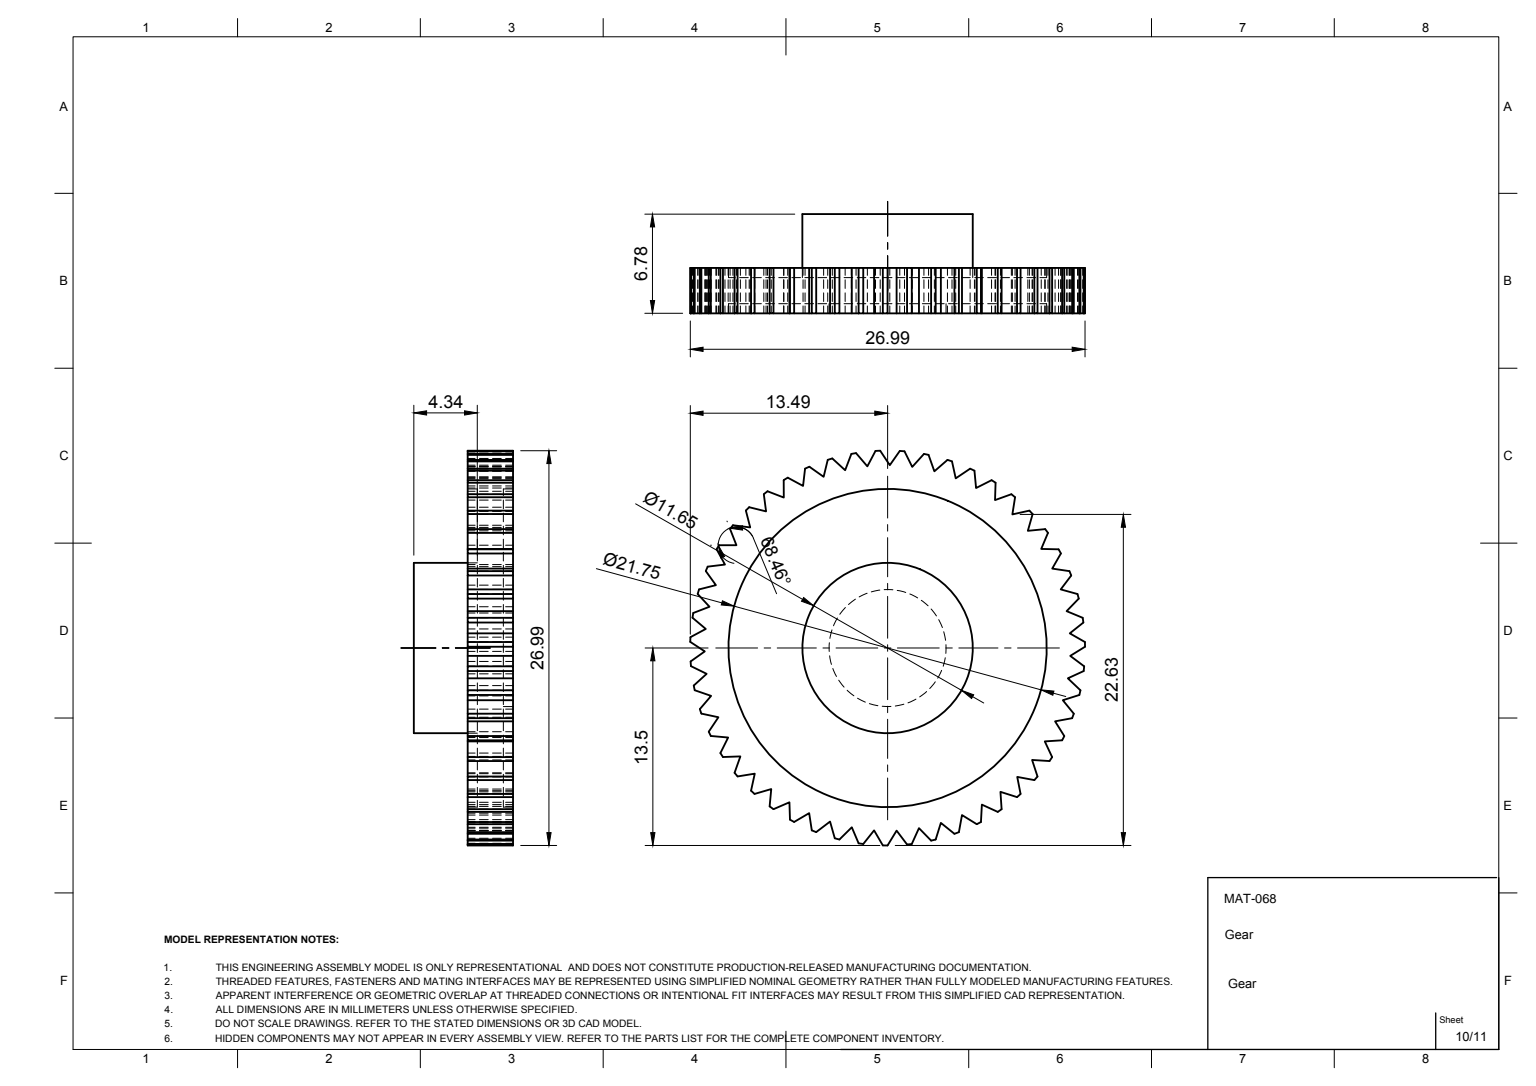
ISO-10303-21;
HEADER;
/* Generated by software containing ST-Developer
 * from STEP Tools, Inc. (www.steptools.com) 
 */

FILE_DESCRIPTION(
/* description */ ('CAx-IF Rec.Pracs.---Representation and Presentation of Product Manufa
cturing Information (PMI)---4.0---2014-10-13'),
/* implementation_level */ '2;1');

FILE_NAME(
/* name */ 'Gear.step',
/* time_stamp */ '2026-10-24T16:53:48-07:00',
/* author */ (''),
/* organization */ (''),
/* preprocessor_version */ 'ST-DEVELOPER v20.2',
/* originating_system */ 'Autodesk Translation Framework v15.17.0.0',
/* authorisation */ '');

FILE_SCHEMA (('AP242_MANAGED_MODEL_BASED_3D_ENGINEERING_MIM_LF { 1 0 10303 442 2 1 4 }'));
ENDSEC;

DATA;
#10=MECHANICAL_DESIGN_GEOMETRIC_PRESENTATION_REPRESENTATION('',(#3497),#107910);
#3477=SHAPE_REPRESENTATION_RELATIONSHIP('SRR','None',#107955,#3487);
#3487=ADVANCED_BREP_SHAPE_REPRESENTATION('',(#3507),#107908);
#3497=STYLED_ITEM('',(#108006),#3507);
#3507=MANIFOLD_SOLID_BREP('Body1',#45545);
#3519=FACE_BOUND('',#9399,.T.);
#3520=FACE_BOUND('',#9401,.T.);
#3521=FACE_BOUND('',#9403,.T.);
#3522=FACE_BOUND('',#9405,.T.);
#3574=PLANE('',#50065);
#3575=PLANE('',#50066);
#3576=PLANE('',#50067);
#3577=PLANE('',#50068);
#3578=PLANE('',#50069);
#3579=PLANE('',#50070);
#3580=PLANE('',#50071);
#3581=PLANE('',#50072);
#3582=PLANE('',#50073);
#3583=PLANE('',#50074);
#3584=PLANE('',#50075);
#3585=PLANE('',#50076);
#3586=PLANE('',#50077);
#3587=PLANE('',#50078);
#3588=PLANE('',#50079);
#3589=PLANE('',#50080);
#3590=PLANE('',#50081);
#3591=PLANE('',#50082);
#3592=PLANE('',#50083);
#3593=PLANE('',#50084);
#3594=PLANE('',#50085);
#3595=PLANE('',#50086);
#3596=PLANE('',#50087);
#3597=PLANE('',#50088);
#3598=PLANE('',#50089);
#3599=PLANE('',#50090);
#3600=PLANE('',#50091);
#3601=PLANE('',#50092);
#3602=PLANE('',#50093);
#3603=PLANE('',#50094);
#3604=PLANE('',#50095);
#3605=PLANE('',#50096);
#3606=PLANE('',#50097);
#3607=PLANE('',#50098);
#3608=PLANE('',#50099);
#3609=PLANE('',#50100);
#3610=PLANE('',#50101);
#3611=PLANE('',#50102);
#3612=PLANE('',#50103);
#3613=PLANE('',#50104);
#3614=PLANE('',#50105);
#3615=PLANE('',#50106);
#3616=PLANE('',#50107);
#3617=PLANE('',#50108);
#3618=PLANE('',#50109);
#3619=PLANE('',#50110);
#3620=PLANE('',#50111);
#3621=PLANE('',#50112);
#3622=PLANE('',#50113);
#3623=PLANE('',#50114);
#3624=PLANE('',#50115);
#3625=PLANE('',#50116);
#3626=PLANE('',#50117);
#3627=PLANE('',#50118);
#3628=PLANE('',#50119);
#3629=PLANE('',#50120);
#3630=PLANE('',#50121);
#3631=PLANE('',#50122);
#3632=PLANE('',#50123);
#3633=PLANE('',#50124);
#3634=PLANE('',#50125);
#3635=PLANE('',#50126);
#3636=PLANE('',#50127);
#3637=PLANE('',#50128);
#3638=PLANE('',#50129);
#3639=PLANE('',#50130);
#3640=PLANE('',#50131);
#3641=PLANE('',#50132);
#3642=PLANE('',#50133);
#3643=PLANE('',#50134);
#3644=PLANE('',#50135);
#3645=PLANE('',#50136);
#3646=PLANE('',#50137);
#3647=PLANE('',#50138);
#3648=PLANE('',#50139);
#3649=PLANE('',#50140);
#3650=PLANE('',#50141);
#3651=PLANE('',#50142);
#3652=PLANE('',#50143);
#3653=PLANE('',#50144);
#3654=PLANE('',#50145);
#3655=PLANE('',#50146);
#3656=PLANE('',#50147);
#3657=PLANE('',#50148);
#3658=PLANE('',#50149);
#3659=PLANE('',#50150);
#3660=PLANE('',#50151);
#3661=PLANE('',#50152);
#3662=PLANE('',#50153);
#3663=PLANE('',#50154);
#3664=PLANE('',#50155);
#3665=PLANE('',#50156);
#3666=PLANE('',#50157);
#3667=PLANE('',#50158);
#3668=PLANE('',#50159);
#3669=PLANE('',#50160);
#3670=PLANE('',#50161);
#3671=PLANE('',#50162);
#3672=PLANE('',#50163);
#3673=PLANE('',#50164);
#3674=PLANE('',#50165);
#3675=PLANE('',#50166);
#3676=PLANE('',#50167);
#3677=PLANE('',#50168);
#3678=PLANE('',#50169);
#3679=PLANE('',#50170);
#3680=PLANE('',#50171);
#3681=PLANE('',#50172);
#6409=FACE_OUTER_BOUND('',#9343,.T.);
#6410=FACE_OUTER_BOUND('',#9344,.T.);
#6411=FACE_OUTER_BOUND('',#9345,.T.);
#6412=FACE_OUTER_BOUND('',#9346,.T.);
#6413=FACE_OUTER_BOUND('',#9347,.T.);
#6414=FACE_OUTER_BOUND('',#9348,.T.);
#6415=FACE_OUTER_BOUND('',#9349,.T.);
#6416=FACE_OUTER_BOUND('',#9350,.T.);
#6417=FACE_OUTER_BOUND('',#9351,.T.);
#6418=FACE_OUTER_BOUND('',#9352,.T.);
#6419=FACE_OUTER_BOUND('',#9353,.T.);
#6420=FACE_OUTER_BOUND('',#9354,.T.);
#6421=FACE_OUTER_BOUND('',#9355,.T.);
#6422=FACE_OUTER_BOUND('',#9356,.T.);
#6423=FACE_OUTER_BOUND('',#9357,.T.);
#6424=FACE_OUTER_BOUND('',#9358,.T.);
#6425=FACE_OUTER_BOUND('',#9359,.T.);
#6426=FACE_OUTER_BOUND('',#9360,.T.);
#6427=FACE_OUTER_BOUND('',#9361,.T.);
#6428=FACE_OUTER_BOUND('',#9362,.T.);
#6429=FACE_OUTER_BOUND('',#9363,.T.);
#6430=FACE_OUTER_BOUND('',#9364,.T.);
#6431=FACE_OUTER_BOUND('',#9365,.T.);
#6432=FACE_OUTER_BOUND('',#9366,.T.);
#6433=FACE_OUTER_BOUND('',#9367,.T.);
#6434=FACE_OUTER_BOUND('',#9368,.T.);
#6435=FACE_OUTER_BOUND('',#9369,.T.);
#6436=FACE_OUTER_BOUND('',#9370,.T.);
#6437=FACE_OUTER_BOUND('',#9371,.T.);
#6438=FACE_OUTER_BOUND('',#9372,.T.);
#6439=FACE_OUTER_BOUND('',#9373,.T.);
#6440=FACE_OUTER_BOUND('',#9374,.T.);
#6441=FACE_OUTER_BOUND('',#9375,.T.);
#6442=FACE_OUTER_BOUND('',#9376,.T.);
#6443=FACE_OUTER_BOUND('',#9377,.T.);
#6444=FACE_OUTER_BOUND('',#9378,.T.);
#6445=FACE_OUTER_BOUND('',#9379,.T.);
#6446=FACE_OUTER_BOUND('',#9380,.T.);
#6447=FACE_OUTER_BOUND('',#9381,.T.);
#6448=FACE_OUTER_BOUND('',#9382,.T.);
#6449=FACE_OUTER_BOUND('',#9383,.T.);
#6450=FACE_OUTER_BOUND('',#9384,.T.);
#6451=FACE_OUTER_BOUND('',#9385,.T.);
#6452=FACE_OUTER_BOUND('',#9386,.T.);
#6453=FACE_OUTER_BOUND('',#9387,.T.);
#6454=FACE_OUTER_BOUND('',#9388,.T.);
#6455=FACE_OUTER_BOUND('',#9389,.T.);
#6456=FACE_OUTER_BOUND('',#9390,.T.);
#6457=FACE_OUTER_BOUND('',#9391,.T.);
#6458=FACE_OUTER_BOUND('',#9392,.T.);
#6459=FACE_OUTER_BOUND('',#9393,.T.);
#6460=FACE_OUTER_BOUND('',#9394,.T.);
#6461=FACE_OUTER_BOUND('',#9395,.T.);
#6462=FACE_OUTER_BOUND('',#9396,.T.);
#6463=FACE_OUTER_BOUND('',#9397,.T.);
#6464=FACE_OUTER_BOUND('',#9398,.T.);
#6465=FACE_OUTER_BOUND('',#9400,.T.);
#6466=FACE_OUTER_BOUND('',#9402,.T.);
#6467=FACE_OUTER_BOUND('',#9404,.T.);
#6468=FACE_OUTER_BOUND('',#9406,.T.);
#6469=FACE_OUTER_BOUND('',#9407,.T.);
#6470=FACE_OUTER_BOUND('',#9408,.T.);
#6471=FACE_OUTER_BOUND('',#9409,.T.);
#6472=FACE_OUTER_BOUND('',#9410,.T.);
#6473=FACE_OUTER_BOUND('',#9411,.T.);
#6474=FACE_OUTER_BOUND('',#9412,.T.);
#6475=FACE_OUTER_BOUND('',#9413,.T.);
#6476=FACE_OUTER_BOUND('',#9414,.T.);
#6477=FACE_OUTER_BOUND('',#9415,.T.);
#6478=FACE_OUTER_BOUND('',#9416,.T.);
#6479=FACE_OUTER_BOUND('',#9417,.T.);
#6480=FACE_OUTER_BOUND('',#9418,.T.);
#6481=FACE_OUTER_BOUND('',#9419,.T.);
#6482=FACE_OUTER_BOUND('',#9420,.T.);
#6483=FACE_OUTER_BOUND('',#9421,.T.);
#6484=FACE_OUTER_BOUND('',#9422,.T.);
#6485=FACE_OUTER_BOUND('',#9423,.T.);
#6486=FACE_OUTER_BOUND('',#9424,.T.);
#6487=FACE_OUTER_BOUND('',#9425,.T.);
#6488=FACE_OUTER_BOUND('',#9426,.T.);
#6489=FACE_OUTER_BOUND('',#9427,.T.);
#6490=FACE_OUTER_BOUND('',#9428,.T.);
#6491=FACE_OUTER_BOUND('',#9429,.T.);
#6492=FACE_OUTER_BOUND('',#9430,.T.);
#6493=FACE_OUTER_BOUND('',#9431,.T.);
#6494=FACE_OUTER_BOUND('',#9432,.T.);
#6495=FACE_OUTER_BOUND('',#9433,.T.);
#6496=FACE_OUTER_BOUND('',#9434,.T.);
#6497=FACE_OUTER_BOUND('',#9435,.T.);
#6498=FACE_OUTER_BOUND('',#9436,.T.);
#6499=FACE_OUTER_BOUND('',#9437,.T.);
#6500=FACE_OUTER_BOUND('',#9438,.T.);
#6501=FACE_OUTER_BOUND('',#9439,.T.);
#6502=FACE_OUTER_BOUND('',#9440,.T.);
#6503=FACE_OUTER_BOUND('',#9441,.T.);
#6504=FACE_OUTER_BOUND('',#9442,.T.);
#6505=FACE_OUTER_BOUND('',#9443,.T.);
#6506=FACE_OUTER_BOUND('',#9444,.T.);
#6507=FACE_OUTER_BOUND('',#9445,.T.);
#6508=FACE_OUTER_BOUND('',#9446,.T.);
#6509=FACE_OUTER_BOUND('',#9447,.T.);
#6510=FACE_OUTER_BOUND('',#9448,.T.);
#6511=FACE_OUTER_BOUND('',#9449,.T.);
#6512=FACE_OUTER_BOUND('',#9450,.T.);
#6513=FACE_OUTER_BOUND('',#9451,.T.);
#6514=FACE_OUTER_BOUND('',#9452,.T.);
#6515=FACE_OUTER_BOUND('',#9453,.T.);
#6516=FACE_OUTER_BOUND('',#9454,.T.);
#6517=FACE_OUTER_BOUND('',#9455,.T.);
#6518=FACE_OUTER_BOUND('',#9456,.T.);
#6519=FACE_OUTER_BOUND('',#9457,.T.);
#6520=FACE_OUTER_BOUND('',#9458,.T.);
#6521=FACE_OUTER_BOUND('',#9459,.T.);
#6522=FACE_OUTER_BOUND('',#9460,.T.);
#6523=FACE_OUTER_BOUND('',#9461,.T.);
#6524=FACE_OUTER_BOUND('',#9462,.T.);
#6525=FACE_OUTER_BOUND('',#9463,.T.);
#6526=FACE_OUTER_BOUND('',#9464,.T.);
#6527=FACE_OUTER_BOUND('',#9465,.T.);
#6528=FACE_OUTER_BOUND('',#9466,.T.);
#6529=FACE_OUTER_BOUND('',#9467,.T.);
#6530=FACE_OUTER_BOUND('',#9468,.T.);
#6531=FACE_OUTER_BOUND('',#9469,.T.);
#6532=FACE_OUTER_BOUND('',#9470,.T.);
#6533=FACE_OUTER_BOUND('',#9471,.T.);
#6534=FACE_OUTER_BOUND('',#9472,.T.);
#6535=FACE_OUTER_BOUND('',#9473,.T.);
#6536=FACE_OUTER_BOUND('',#9474,.T.);
#6537=FACE_OUTER_BOUND('',#9475,.T.);
#6538=FACE_OUTER_BOUND('',#9476,.T.);
#6539=FACE_OUTER_BOUND('',#9477,.T.);
#6540=FACE_OUTER_BOUND('',#9478,.T.);
#6541=FACE_OUTER_BOUND('',#9479,.T.);
#6542=FACE_OUTER_BOUND('',#9480,.T.);
#6543=FACE_OUTER_BOUND('',#9481,.T.);
#6544=FACE_OUTER_BOUND('',#9482,.T.);
#6545=FACE_OUTER_BOUND('',#9483,.T.);
#6546=FACE_OUTER_BOUND('',#9484,.T.);
#6547=FACE_OUTER_BOUND('',#9485,.T.);
#6548=FACE_OUTER_BOUND('',#9486,.T.);
#6549=FACE_OUTER_BOUND('',#9487,.T.);
#6550=FACE_OUTER_BOUND('',#9488,.T.);
#6551=FACE_OUTER_BOUND('',#9489,.T.);
#6552=FACE_OUTER_BOUND('',#9490,.T.);
#6553=FACE_OUTER_BOUND('',#9491,.T.);
#6554=FACE_OUTER_BOUND('',#9492,.T.);
#6555=FACE_OUTER_BOUND('',#9493,.T.);
#6556=FACE_OUTER_BOUND('',#9494,.T.);
#6557=FACE_OUTER_BOUND('',#9495,.T.);
#6558=FACE_OUTER_BOUND('',#9496,.T.);
#6559=FACE_OUTER_BOUND('',#9497,.T.);
#6560=FACE_OUTER_BOUND('',#9498,.T.);
#6561=FACE_OUTER_BOUND('',#9499,.T.);
#6562=FACE_OUTER_BOUND('',#9500,.T.);
#6563=FACE_OUTER_BOUND('',#9501,.T.);
#6564=FACE_OUTER_BOUND('',#9502,.T.);
#6565=FACE_OUTER_BOUND('',#9503,.T.);
#6566=FACE_OUTER_BOUND('',#9504,.T.);
#6567=FACE_OUTER_BOUND('',#9505,.T.);
#6568=FACE_OUTER_BOUND('',#9506,.T.);
#6569=FACE_OUTER_BOUND('',#9507,.T.);
#6570=FACE_OUTER_BOUND('',#9508,.T.);
#6571=FACE_OUTER_BOUND('',#9509,.T.);
#9343=EDGE_LOOP('',(#40412,#40413,#40414,#40415));
#9344=EDGE_LOOP('',(#40416,#40417,#40418,#40419));
#9345=EDGE_LOOP('',(#40420,#40421,#40422,#40423));
#9346=EDGE_LOOP('',(#40424,#40425,#40426,#40427));
#9347=EDGE_LOOP('',(#40428,#40429,#40430,#40431));
#9348=EDGE_LOOP('',(#40432,#40433,#40434,#40435));
#9349=EDGE_LOOP('',(#40436,#40437,#40438,#40439));
#9350=EDGE_LOOP('',(#40440,#40441,#40442,#40443));
#9351=EDGE_LOOP('',(#40444,#40445,#40446,#40447));
#9352=EDGE_LOOP('',(#40448,#40449,#40450,#40451));
#9353=EDGE_LOOP('',(#40452,#40453,#40454,#40455));
#9354=EDGE_LOOP('',(#40456,#40457,#40458,#40459));
#9355=EDGE_LOOP('',(#40460,#40461,#40462,#40463));
#9356=EDGE_LOOP('',(#40464,#40465,#40466,#40467));
#9357=EDGE_LOOP('',(#40468,#40469,#40470,#40471));
#9358=EDGE_LOOP('',(#40472,#40473,#40474,#40475));
#9359=EDGE_LOOP('',(#40476,#40477,#40478,#40479));
#9360=EDGE_LOOP('',(#40480,#40481,#40482,#40483));
#9361=EDGE_LOOP('',(#40484,#40485,#40486,#40487));
#9362=EDGE_LOOP('',(#40488,#40489,#40490,#40491));
#9363=EDGE_LOOP('',(#40492,#40493,#40494,#40495));
#9364=EDGE_LOOP('',(#40496,#40497,#40498,#40499));
#9365=EDGE_LOOP('',(#40500,#40501,#40502,#40503));
#9366=EDGE_LOOP('',(#40504,#40505,#40506,#40507));
#9367=EDGE_LOOP('',(#40508,#40509,#40510,#40511));
#9368=EDGE_LOOP('',(#40512,#40513,#40514,#40515));
#9369=EDGE_LOOP('',(#40516,#40517,#40518,#40519));
#9370=EDGE_LOOP('',(#40520,#40521,#40522,#40523));
#9371=EDGE_LOOP('',(#40524,#40525,#40526,#40527));
#9372=EDGE_LOOP('',(#40528,#40529,#40530,#40531));
#9373=EDGE_LOOP('',(#40532,#40533,#40534,#40535));
#9374=EDGE_LOOP('',(#40536,#40537,#40538,#40539));
#9375=EDGE_LOOP('',(#40540,#40541,#40542,#40543));
#9376=EDGE_LOOP('',(#40544,#40545,#40546,#40547));
#9377=EDGE_LOOP('',(#40548,#40549,#40550,#40551));
#9378=EDGE_LOOP('',(#40552,#40553,#40554,#40555));
#9379=EDGE_LOOP('',(#40556,#40557,#40558,#40559));
#9380=EDGE_LOOP('',(#40560,#40561,#40562,#40563));
#9381=EDGE_LOOP('',(#40564,#40565,#40566,#40567));
#9382=EDGE_LOOP('',(#40568,#40569,#40570,#40571));
#9383=EDGE_LOOP('',(#40572,#40573,#40574,#40575));
#9384=EDGE_LOOP('',(#40576,#40577,#40578,#40579));
#9385=EDGE_LOOP('',(#40580,#40581,#40582,#40583));
#9386=EDGE_LOOP('',(#40584,#40585,#40586,#40587));
#9387=EDGE_LOOP('',(#40588,#40589,#40590,#40591));
#9388=EDGE_LOOP('',(#40592,#40593,#40594,#40595));
#9389=EDGE_LOOP('',(#40596,#40597,#40598,#40599));
#9390=EDGE_LOOP('',(#40600,#40601,#40602,#40603));
#9391=EDGE_LOOP('',(#40604,#40605,#40606,#40607));
#9392=EDGE_LOOP('',(#40608,#40609,#40610,#40611));
#9393=EDGE_LOOP('',(#40612,#40613,#40614,#40615));
#9394=EDGE_LOOP('',(#40616,#40617,#40618,#40619));
#9395=EDGE_LOOP('',(#40620,#40621,#40622,#40623));
#9396=EDGE_LOOP('',(#40624,#40625,#40626,#40627));
#9397=EDGE_LOOP('',(#40628,#40629,#40630,#40631));
#9398=EDGE_LOOP('',(#40632,#40633,#40634,#40635,#40636,#40637,#40638,#40639,
#40640,#40641,#40642,#40643,#40644,#40645,#40646,#40647,#40648,#40649,#40650,
#40651,#40652,#40653,#40654,#40655,#40656,#40657,#40658,#40659,#40660,#40661,
#40662,#40663,#40664,#40665,#40666,#40667,#40668,#40669,#40670,#40671,#40672,
#40673,#40674,#40675,#40676,#40677,#40678,#40679,#40680,#40681,#40682,#40683,
#40684,#40685,#40686,#40687,#40688,#40689,#40690,#40691,#40692,#40693,#40694,
#40695,#40696,#40697,#40698,#40699,#40700,#40701,#40702,#40703,#40704,#40705,
#40706,#40707,#40708,#40709,#40710,#40711,#40712,#40713,#40714,#40715,#40716,
#40717,#40718,#40719,#40720,#40721,#40722,#40723,#40724,#40725,#40726,#40727,
#40728,#40729,#40730,#40731,#40732,#40733,#40734,#40735,#40736,#40737,#40738,
#40739,#40740,#40741,#40742,#40743,#40744,#40745,#40746,#40747,#40748,#40749,
#40750,#40751,#40752,#40753,#40754,#40755,#40756,#40757,#40758,#40759,#40760,
#40761,#40762,#40763,#40764,#40765,#40766,#40767,#40768,#40769,#40770,#40771,
#40772,#40773,#40774,#40775,#40776,#40777,#40778,#40779,#40780,#40781,#40782,
#40783,#40784));
#9399=EDGE_LOOP('',(#40785));
#9400=EDGE_LOOP('',(#40786,#40787,#40788,#40789,#40790,#40791,#40792,#40793,
#40794,#40795,#40796,#40797,#40798,#40799,#40800,#40801,#40802,#40803,#40804,
#40805,#40806,#40807,#40808,#40809,#40810,#40811,#40812,#40813,#40814,#40815,
#40816,#40817,#40818,#40819,#40820,#40821,#40822,#40823,#40824,#40825,#40826,
#40827,#40828,#40829,#40830,#40831,#40832,#40833,#40834,#40835,#40836,#40837,
#40838,#40839,#40840,#40841,#40842,#40843,#40844,#40845,#40846,#40847,#40848,
#40849,#40850,#40851,#40852,#40853,#40854,#40855,#40856,#40857,#40858,#40859,
#40860,#40861,#40862,#40863,#40864,#40865,#40866,#40867,#40868,#40869,#40870,
#40871,#40872,#40873,#40874,#40875,#40876,#40877,#40878,#40879,#40880,#40881,
#40882,#40883,#40884,#40885,#40886,#40887,#40888,#40889,#40890,#40891,#40892,
#40893,#40894,#40895,#40896,#40897,#40898,#40899,#40900,#40901,#40902,#40903,
#40904,#40905,#40906,#40907,#40908,#40909,#40910,#40911,#40912,#40913,#40914,
#40915,#40916,#40917,#40918,#40919,#40920,#40921,#40922,#40923,#40924,#40925,
#40926,#40927,#40928,#40929,#40930,#40931,#40932,#40933,#40934,#40935,#40936,
#40937,#40938));
#9401=EDGE_LOOP('',(#40939));
#9402=EDGE_LOOP('',(#40940));
#9403=EDGE_LOOP('',(#40941));
#9404=EDGE_LOOP('',(#40942));
#9405=EDGE_LOOP('',(#40943));
#9406=EDGE_LOOP('',(#40944));
#9407=EDGE_LOOP('',(#40945));
#9408=EDGE_LOOP('',(#40946,#40947,#40948,#40949));
#9409=EDGE_LOOP('',(#40950,#40951,#40952,#40953));
#9410=EDGE_LOOP('',(#40954,#40955,#40956,#40957));
#9411=EDGE_LOOP('',(#40958,#40959,#40960,#40961));
#9412=EDGE_LOOP('',(#40962,#40963,#40964,#40965));
#9413=EDGE_LOOP('',(#40966,#40967,#40968,#40969));
#9414=EDGE_LOOP('',(#40970,#40971,#40972,#40973));
#9415=EDGE_LOOP('',(#40974,#40975,#40976,#40977));
#9416=EDGE_LOOP('',(#40978,#40979,#40980,#40981));
#9417=EDGE_LOOP('',(#40982,#40983,#40984,#40985));
#9418=EDGE_LOOP('',(#40986,#40987,#40988,#40989));
#9419=EDGE_LOOP('',(#40990,#40991,#40992,#40993));
#9420=EDGE_LOOP('',(#40994,#40995,#40996,#40997));
#9421=EDGE_LOOP('',(#40998,#40999,#41000,#41001));
#9422=EDGE_LOOP('',(#41002,#41003,#41004,#41005));
#9423=EDGE_LOOP('',(#41006,#41007,#41008,#41009));
#9424=EDGE_LOOP('',(#41010,#41011,#41012,#41013));
#9425=EDGE_LOOP('',(#41014,#41015,#41016,#41017));
#9426=EDGE_LOOP('',(#41018,#41019,#41020,#41021));
#9427=EDGE_LOOP('',(#41022,#41023,#41024,#41025));
#9428=EDGE_LOOP('',(#41026,#41027,#41028,#41029));
#9429=EDGE_LOOP('',(#41030,#41031,#41032,#41033));
#9430=EDGE_LOOP('',(#41034,#41035,#41036,#41037));
#9431=EDGE_LOOP('',(#41038,#41039,#41040,#41041));
#9432=EDGE_LOOP('',(#41042,#41043,#41044,#41045));
#9433=EDGE_LOOP('',(#41046,#41047,#41048,#41049));
#9434=EDGE_LOOP('',(#41050,#41051,#41052,#41053));
#9435=EDGE_LOOP('',(#41054,#41055,#41056,#41057));
#9436=EDGE_LOOP('',(#41058,#41059,#41060,#41061));
#9437=EDGE_LOOP('',(#41062,#41063,#41064,#41065));
#9438=EDGE_LOOP('',(#41066,#41067,#41068,#41069));
#9439=EDGE_LOOP('',(#41070,#41071,#41072,#41073));
#9440=EDGE_LOOP('',(#41074,#41075,#41076,#41077));
#9441=EDGE_LOOP('',(#41078,#41079,#41080,#41081));
#9442=EDGE_LOOP('',(#41082,#41083,#41084,#41085));
#9443=EDGE_LOOP('',(#41086,#41087,#41088,#41089));
#9444=EDGE_LOOP('',(#41090,#41091,#41092,#41093));
#9445=EDGE_LOOP('',(#41094,#41095,#41096,#41097));
#9446=EDGE_LOOP('',(#41098,#41099,#41100,#41101));
#9447=EDGE_LOOP('',(#41102,#41103,#41104,#41105));
#9448=EDGE_LOOP('',(#41106,#41107,#41108,#41109));
#9449=EDGE_LOOP('',(#41110,#41111,#41112,#41113));
#9450=EDGE_LOOP('',(#41114,#41115,#41116,#41117));
#9451=EDGE_LOOP('',(#41118,#41119,#41120,#41121));
#9452=EDGE_LOOP('',(#41122,#41123,#41124,#41125));
#9453=EDGE_LOOP('',(#41126,#41127,#41128,#41129));
#9454=EDGE_LOOP('',(#41130,#41131,#41132,#41133));
#9455=EDGE_LOOP('',(#41134,#41135,#41136,#41137));
#9456=EDGE_LOOP('',(#41138,#41139,#41140,#41141));
#9457=EDGE_LOOP('',(#41142,#41143,#41144,#41145));
#9458=EDGE_LOOP('',(#41146,#41147,#41148,#41149));
#9459=EDGE_LOOP('',(#41150,#41151,#41152,#41153));
#9460=EDGE_LOOP('',(#41154,#41155,#41156,#41157));
#9461=EDGE_LOOP('',(#41158,#41159,#41160,#41161));
#9462=EDGE_LOOP('',(#41162,#41163,#41164,#41165));
#9463=EDGE_LOOP('',(#41166,#41167,#41168,#41169));
#9464=EDGE_LOOP('',(#41170,#41171,#41172,#41173));
#9465=EDGE_LOOP('',(#41174,#41175,#41176,#41177));
#9466=EDGE_LOOP('',(#41178,#41179,#41180,#41181));
#9467=EDGE_LOOP('',(#41182,#41183,#41184,#41185));
#9468=EDGE_LOOP('',(#41186,#41187,#41188,#41189));
#9469=EDGE_LOOP('',(#41190,#41191,#41192,#41193));
#9470=EDGE_LOOP('',(#41194,#41195,#41196,#41197));
#9471=EDGE_LOOP('',(#41198,#41199,#41200,#41201));
#9472=EDGE_LOOP('',(#41202,#41203,#41204,#41205));
#9473=EDGE_LOOP('',(#41206,#41207,#41208,#41209));
#9474=EDGE_LOOP('',(#41210,#41211,#41212,#41213));
#9475=EDGE_LOOP('',(#41214,#41215,#41216,#41217));
#9476=EDGE_LOOP('',(#41218,#41219,#41220,#41221));
#9477=EDGE_LOOP('',(#41222,#41223,#41224,#41225));
#9478=EDGE_LOOP('',(#41226,#41227,#41228,#41229));
#9479=EDGE_LOOP('',(#41230,#41231,#41232,#41233));
#9480=EDGE_LOOP('',(#41234,#41235,#41236,#41237));
#9481=EDGE_LOOP('',(#41238,#41239,#41240,#41241));
#9482=EDGE_LOOP('',(#41242,#41243,#41244,#41245));
#9483=EDGE_LOOP('',(#41246,#41247,#41248,#41249));
#9484=EDGE_LOOP('',(#41250,#41251,#41252,#41253));
#9485=EDGE_LOOP('',(#41254,#41255,#41256,#41257));
#9486=EDGE_LOOP('',(#41258,#41259,#41260,#41261));
#9487=EDGE_LOOP('',(#41262,#41263,#41264,#41265));
#9488=EDGE_LOOP('',(#41266,#41267,#41268,#41269));
#9489=EDGE_LOOP('',(#41270,#41271,#41272,#41273));
#9490=EDGE_LOOP('',(#41274,#41275,#41276,#41277));
#9491=EDGE_LOOP('',(#41278,#41279,#41280,#41281));
#9492=EDGE_LOOP('',(#41282,#41283,#41284,#41285));
#9493=EDGE_LOOP('',(#41286,#41287,#41288,#41289));
#9494=EDGE_LOOP('',(#41290,#41291,#41292,#41293));
#9495=EDGE_LOOP('',(#41294,#41295,#41296,#41297));
#9496=EDGE_LOOP('',(#41298,#41299,#41300,#41301));
#9497=EDGE_LOOP('',(#41302,#41303,#41304,#41305));
#9498=EDGE_LOOP('',(#41306,#41307,#41308,#41309));
#9499=EDGE_LOOP('',(#41310,#41311,#41312,#41313));
#9500=EDGE_LOOP('',(#41314,#41315,#41316,#41317));
#9501=EDGE_LOOP('',(#41318,#41319,#41320,#41321));
#9502=EDGE_LOOP('',(#41322,#41323,#41324,#41325));
#9503=EDGE_LOOP('',(#41326,#41327,#41328,#41329));
#9504=EDGE_LOOP('',(#41330,#41331,#41332,#41333));
#9505=EDGE_LOOP('',(#41334,#41335,#41336,#41337));
#9506=EDGE_LOOP('',(#41338,#41339,#41340,#41341));
#9507=EDGE_LOOP('',(#41342,#41343,#41344,#41345));
#9508=EDGE_LOOP('',(#41346,#41347,#41348,#41349));
#9509=EDGE_LOOP('',(#41350,#41351,#41352,#41353));
#11044=LINE('',#106266,#13028);
#11045=LINE('',#106272,#13029);
#11046=LINE('',#106278,#13030);
#11047=LINE('',#106284,#13031);
#11048=LINE('',#106289,#13032);
#11049=LINE('',#106293,#13033);
#11050=LINE('',#106298,#13034);
#11051=LINE('',#106302,#13035);
#11052=LINE('',#106307,#13036);
#11053=LINE('',#106311,#13037);
#11054=LINE('',#106316,#13038);
#11055=LINE('',#106320,#13039);
#11056=LINE('',#106325,#13040);
#11057=LINE('',#106329,#13041);
#11058=LINE('',#106334,#13042);
#11059=LINE('',#106338,#13043);
#11060=LINE('',#106343,#13044);
#11061=LINE('',#106347,#13045);
#11062=LINE('',#106352,#13046);
#11063=LINE('',#106356,#13047);
#11064=LINE('',#106361,#13048);
#11065=LINE('',#106365,#13049);
#11066=LINE('',#106370,#13050);
#11067=LINE('',#106374,#13051);
#11068=LINE('',#106379,#13052);
#11069=LINE('',#106383,#13053);
#11070=LINE('',#106388,#13054);
#11071=LINE('',#106392,#13055);
#11072=LINE('',#106397,#13056);
#11073=LINE('',#106401,#13057);
#11074=LINE('',#106406,#13058);
#11075=LINE('',#106410,#13059);
#11076=LINE('',#106415,#13060);
#11077=LINE('',#106419,#13061);
#11078=LINE('',#106424,#13062);
#11079=LINE('',#106428,#13063);
#11080=LINE('',#106433,#13064);
#11081=LINE('',#106437,#13065);
#11082=LINE('',#106442,#13066);
#11083=LINE('',#106446,#13067);
#11084=LINE('',#106451,#13068);
#11085=LINE('',#106455,#13069);
#11086=LINE('',#106460,#13070);
#11087=LINE('',#106464,#13071);
#11088=LINE('',#106469,#13072);
#11089=LINE('',#106473,#13073);
#11090=LINE('',#106478,#13074);
#11091=LINE('',#106482,#13075);
#11092=LINE('',#106487,#13076);
#11093=LINE('',#106491,#13077);
#11094=LINE('',#106496,#13078);
#11095=LINE('',#106500,#13079);
#11096=LINE('',#106505,#13080);
#11097=LINE('',#106509,#13081);
#11098=LINE('',#106514,#13082);
#11099=LINE('',#106518,#13083);
#11100=LINE('',#106523,#13084);
#11101=LINE('',#106527,#13085);
#11102=LINE('',#106532,#13086);
#11103=LINE('',#106536,#13087);
#11104=LINE('',#106541,#13088);
#11105=LINE('',#106545,#13089);
#11106=LINE('',#106550,#13090);
#11107=LINE('',#106554,#13091);
#11108=LINE('',#106559,#13092);
#11109=LINE('',#106563,#13093);
#11110=LINE('',#106568,#13094);
#11111=LINE('',#106572,#13095);
#11112=LINE('',#106577,#13096);
#11113=LINE('',#106581,#13097);
#11114=LINE('',#106586,#13098);
#11115=LINE('',#106590,#13099);
#11116=LINE('',#106595,#13100);
#11117=LINE('',#106599,#13101);
#11118=LINE('',#106604,#13102);
#11119=LINE('',#106608,#13103);
#11120=LINE('',#106613,#13104);
#11121=LINE('',#106617,#13105);
#11122=LINE('',#106622,#13106);
#11123=LINE('',#106626,#13107);
#11124=LINE('',#106631,#13108);
#11125=LINE('',#106635,#13109);
#11126=LINE('',#106640,#13110);
#11127=LINE('',#106644,#13111);
#11128=LINE('',#106649,#13112);
#11129=LINE('',#106653,#13113);
#11130=LINE('',#106658,#13114);
#11131=LINE('',#106662,#13115);
#11132=LINE('',#106667,#13116);
#11133=LINE('',#106671,#13117);
#11134=LINE('',#106676,#13118);
#11135=LINE('',#106680,#13119);
#11136=LINE('',#106685,#13120);
#11137=LINE('',#106689,#13121);
#11138=LINE('',#106694,#13122);
#11139=LINE('',#106698,#13123);
#11140=LINE('',#106703,#13124);
#11141=LINE('',#106707,#13125);
#11142=LINE('',#106712,#13126);
#11143=LINE('',#106716,#13127);
#11144=LINE('',#106721,#13128);
#11145=LINE('',#106725,#13129);
#11146=LINE('',#106730,#13130);
#11147=LINE('',#106734,#13131);
#11148=LINE('',#106739,#13132);
#11149=LINE('',#106743,#13133);
#11150=LINE('',#106747,#13134);
#11151=LINE('',#106748,#13135);
#11152=LINE('',#106750,#13136);
#11153=LINE('',#106751,#13137);
#11154=LINE('',#106753,#13138);
#11155=LINE('',#106754,#13139);
#11156=LINE('',#106756,#13140);
#11157=LINE('',#106757,#13141);
#11158=LINE('',#106759,#13142);
#11159=LINE('',#106760,#13143);
#11160=LINE('',#106762,#13144);
#11161=LINE('',#106763,#13145);
#11162=LINE('',#106765,#13146);
#11163=LINE('',#106766,#13147);
#11164=LINE('',#106768,#13148);
#11165=LINE('',#106769,#13149);
#11166=LINE('',#106771,#13150);
#11167=LINE('',#106772,#13151);
#11168=LINE('',#106774,#13152);
#11169=LINE('',#106775,#13153);
#11170=LINE('',#106777,#13154);
#11171=LINE('',#106778,#13155);
#11172=LINE('',#106780,#13156);
#11173=LINE('',#106781,#13157);
#11174=LINE('',#106783,#13158);
#11175=LINE('',#106784,#13159);
#11176=LINE('',#106786,#13160);
#11177=LINE('',#106787,#13161);
#11178=LINE('',#106789,#13162);
#11179=LINE('',#106790,#13163);
#11180=LINE('',#106792,#13164);
#11181=LINE('',#106793,#13165);
#11182=LINE('',#106795,#13166);
#11183=LINE('',#106796,#13167);
#11184=LINE('',#106798,#13168);
#11185=LINE('',#106799,#13169);
#11186=LINE('',#106801,#13170);
#11187=LINE('',#106802,#13171);
#11188=LINE('',#106804,#13172);
#11189=LINE('',#106805,#13173);
#11190=LINE('',#106807,#13174);
#11191=LINE('',#106808,#13175);
#11192=LINE('',#106810,#13176);
#11193=LINE('',#106811,#13177);
#11194=LINE('',#106813,#13178);
#11195=LINE('',#106814,#13179);
#11196=LINE('',#106816,#13180);
#11197=LINE('',#106817,#13181);
#11198=LINE('',#106819,#13182);
#11199=LINE('',#106820,#13183);
#11200=LINE('',#106822,#13184);
#11201=LINE('',#106823,#13185);
#11202=LINE('',#106825,#13186);
#11203=LINE('',#106826,#13187);
#11204=LINE('',#106828,#13188);
#11205=LINE('',#106829,#13189);
#11206=LINE('',#106831,#13190);
#11207=LINE('',#106832,#13191);
#11208=LINE('',#106834,#13192);
#11209=LINE('',#106835,#13193);
#11210=LINE('',#106837,#13194);
#11211=LINE('',#106838,#13195);
#11212=LINE('',#106840,#13196);
#11213=LINE('',#106841,#13197);
#11214=LINE('',#106843,#13198);
#11215=LINE('',#106844,#13199);
#11216=LINE('',#106846,#13200);
#11217=LINE('',#106847,#13201);
#11218=LINE('',#106849,#13202);
#11219=LINE('',#106850,#13203);
#11220=LINE('',#106852,#13204);
#11221=LINE('',#106853,#13205);
#11222=LINE('',#106855,#13206);
#11223=LINE('',#106856,#13207);
#11224=LINE('',#106858,#13208);
#11225=LINE('',#106859,#13209);
#11226=LINE('',#106861,#13210);
#11227=LINE('',#106862,#13211);
#11228=LINE('',#106864,#13212);
#11229=LINE('',#106865,#13213);
#11230=LINE('',#106867,#13214);
#11231=LINE('',#106868,#13215);
#11232=LINE('',#106870,#13216);
#11233=LINE('',#106871,#13217);
#11234=LINE('',#106873,#13218);
#11235=LINE('',#106874,#13219);
#11236=LINE('',#106876,#13220);
#11237=LINE('',#106877,#13221);
#11238=LINE('',#106879,#13222);
#11239=LINE('',#106880,#13223);
#11240=LINE('',#106882,#13224);
#11241=LINE('',#106883,#13225);
#11242=LINE('',#106885,#13226);
#11243=LINE('',#106886,#13227);
#11244=LINE('',#106888,#13228);
#11245=LINE('',#106889,#13229);
#11246=LINE('',#106891,#13230);
#11247=LINE('',#106892,#13231);
#11248=LINE('',#106894,#13232);
#11249=LINE('',#106895,#13233);
#11250=LINE('',#106897,#13234);
#11251=LINE('',#106898,#13235);
#11252=LINE('',#106901,#13236);
#11253=LINE('',#106902,#13237);
#11254=LINE('',#106904,#13238);
#11255=LINE('',#106905,#13239);
#11256=LINE('',#106907,#13240);
#11257=LINE('',#106908,#13241);
#11258=LINE('',#106910,#13242);
#11259=LINE('',#106911,#13243);
#11260=LINE('',#106913,#13244);
#11261=LINE('',#106914,#13245);
#11262=LINE('',#106916,#13246);
#11263=LINE('',#106917,#13247);
#11264=LINE('',#106919,#13248);
#11265=LINE('',#106920,#13249);
#11266=LINE('',#106922,#13250);
#11267=LINE('',#106923,#13251);
#11268=LINE('',#106925,#13252);
#11269=LINE('',#106926,#13253);
#11270=LINE('',#106928,#13254);
#11271=LINE('',#106929,#13255);
#11272=LINE('',#106931,#13256);
#11273=LINE('',#106932,#13257);
#11274=LINE('',#106934,#13258);
#11275=LINE('',#106935,#13259);
#11276=LINE('',#106937,#13260);
#11277=LINE('',#106938,#13261);
#11278=LINE('',#106940,#13262);
#11279=LINE('',#106941,#13263);
#11280=LINE('',#106943,#13264);
#11281=LINE('',#106944,#13265);
#11282=LINE('',#106946,#13266);
#11283=LINE('',#106947,#13267);
#11284=LINE('',#106949,#13268);
#11285=LINE('',#106950,#13269);
#11286=LINE('',#106952,#13270);
#11287=LINE('',#106953,#13271);
#11288=LINE('',#106955,#13272);
#11289=LINE('',#106956,#13273);
#11290=LINE('',#106958,#13274);
#11291=LINE('',#106959,#13275);
#11292=LINE('',#106961,#13276);
#11293=LINE('',#106962,#13277);
#11294=LINE('',#106964,#13278);
#11295=LINE('',#106965,#13279);
#11296=LINE('',#106967,#13280);
#11297=LINE('',#106968,#13281);
#11298=LINE('',#106970,#13282);
#11299=LINE('',#106971,#13283);
#11300=LINE('',#106973,#13284);
#11301=LINE('',#106974,#13285);
#11302=LINE('',#106976,#13286);
#11303=LINE('',#106977,#13287);
#11304=LINE('',#106979,#13288);
#11305=LINE('',#106980,#13289);
#11306=LINE('',#106982,#13290);
#11307=LINE('',#106983,#13291);
#11308=LINE('',#106985,#13292);
#11309=LINE('',#106986,#13293);
#11310=LINE('',#106988,#13294);
#11311=LINE('',#106989,#13295);
#11312=LINE('',#106991,#13296);
#11313=LINE('',#106992,#13297);
#11314=LINE('',#106994,#13298);
#11315=LINE('',#106995,#13299);
#11316=LINE('',#106997,#13300);
#11317=LINE('',#106998,#13301);
#11318=LINE('',#107000,#13302);
#11319=LINE('',#107001,#13303);
#11320=LINE('',#107003,#13304);
#11321=LINE('',#107004,#13305);
#11322=LINE('',#107006,#13306);
#11323=LINE('',#107007,#13307);
#11324=LINE('',#107009,#13308);
#11325=LINE('',#107010,#13309);
#11326=LINE('',#107012,#13310);
#11327=LINE('',#107013,#13311);
#11328=LINE('',#107015,#13312);
#11329=LINE('',#107016,#13313);
#11330=LINE('',#107018,#13314);
#11331=LINE('',#107019,#13315);
#11332=LINE('',#107021,#13316);
#11333=LINE('',#107022,#13317);
#11334=LINE('',#107024,#13318);
#11335=LINE('',#107025,#13319);
#11336=LINE('',#107027,#13320);
#11337=LINE('',#107028,#13321);
#11338=LINE('',#107030,#13322);
#11339=LINE('',#107031,#13323);
#11340=LINE('',#107033,#13324);
#11341=LINE('',#107034,#13325);
#11342=LINE('',#107036,#13326);
#11343=LINE('',#107037,#13327);
#11344=LINE('',#107039,#13328);
#11345=LINE('',#107040,#13329);
#11346=LINE('',#107042,#13330);
#11347=LINE('',#107043,#13331);
#11348=LINE('',#107045,#13332);
#11349=LINE('',#107046,#13333);
#11350=LINE('',#107048,#13334);
#11351=LINE('',#107049,#13335);
#11352=LINE('',#107051,#13336);
#11353=LINE('',#107052,#13337);
#11354=LINE('',#107058,#13338);
#11355=LINE('',#107061,#13339);
#11356=LINE('',#107064,#13340);
#11357=LINE('',#107067,#13341);
#11358=LINE('',#107070,#13342);
#11359=LINE('',#107073,#13343);
#11360=LINE('',#107076,#13344);
#11361=LINE('',#107079,#13345);
#11362=LINE('',#107082,#13346);
#11363=LINE('',#107085,#13347);
#11364=LINE('',#107088,#13348);
#11365=LINE('',#107091,#13349);
#11366=LINE('',#107094,#13350);
#11367=LINE('',#107097,#13351);
#11368=LINE('',#107100,#13352);
#11369=LINE('',#107103,#13353);
#11370=LINE('',#107106,#13354);
#11371=LINE('',#107109,#13355);
#11372=LINE('',#107112,#13356);
#11373=LINE('',#107115,#13357);
#11374=LINE('',#107118,#13358);
#11375=LINE('',#107121,#13359);
#11376=LINE('',#107124,#13360);
#11377=LINE('',#107127,#13361);
#11378=LINE('',#107130,#13362);
#11379=LINE('',#107133,#13363);
#11380=LINE('',#107136,#13364);
#11381=LINE('',#107139,#13365);
#11382=LINE('',#107142,#13366);
#11383=LINE('',#107145,#13367);
#11384=LINE('',#107148,#13368);
#11385=LINE('',#107151,#13369);
#11386=LINE('',#107154,#13370);
#11387=LINE('',#107157,#13371);
#11388=LINE('',#107160,#13372);
#11389=LINE('',#107163,#13373);
#11390=LINE('',#107166,#13374);
#11391=LINE('',#107169,#13375);
#11392=LINE('',#107172,#13376);
#11393=LINE('',#107175,#13377);
#11394=LINE('',#107178,#13378);
#11395=LINE('',#107181,#13379);
#11396=LINE('',#107184,#13380);
#11397=LINE('',#107187,#13381);
#11398=LINE('',#107190,#13382);
#11399=LINE('',#107193,#13383);
#11400=LINE('',#107196,#13384);
#11401=LINE('',#107199,#13385);
#11402=LINE('',#107202,#13386);
#11403=LINE('',#107205,#13387);
#11404=LINE('',#107208,#13388);
#13028=VECTOR('',#60269,0.004);
#13029=VECTOR('',#60276,0.005825);
#13030=VECTOR('',#60283,0.010875);
#13031=VECTOR('',#60290,0.010875);
#13032=VECTOR('',#60295,1.);
#13033=VECTOR('',#60298,1.);
#13034=VECTOR('',#60303,1.);
#13035=VECTOR('',#60306,1.);
#13036=VECTOR('',#60311,1.);
#13037=VECTOR('',#60314,1.);
#13038=VECTOR('',#60319,1.);
#13039=VECTOR('',#60322,1.);
#13040=VECTOR('',#60327,1.);
#13041=VECTOR('',#60330,1.);
#13042=VECTOR('',#60335,1.);
#13043=VECTOR('',#60338,1.);
#13044=VECTOR('',#60343,1.);
#13045=VECTOR('',#60346,1.);
#13046=VECTOR('',#60351,1.);
#13047=VECTOR('',#60354,1.);
#13048=VECTOR('',#60359,1.);
#13049=VECTOR('',#60362,1.);
#13050=VECTOR('',#60367,1.);
#13051=VECTOR('',#60370,1.);
#13052=VECTOR('',#60375,1.);
#13053=VECTOR('',#60378,1.);
#13054=VECTOR('',#60383,1.);
#13055=VECTOR('',#60386,1.);
#13056=VECTOR('',#60391,1.);
#13057=VECTOR('',#60394,1.);
#13058=VECTOR('',#60399,1.);
#13059=VECTOR('',#60402,1.);
#13060=VECTOR('',#60407,1.);
#13061=VECTOR('',#60410,1.);
#13062=VECTOR('',#60415,1.);
#13063=VECTOR('',#60418,1.);
#13064=VECTOR('',#60423,1.);
#13065=VECTOR('',#60426,1.);
#13066=VECTOR('',#60431,1.);
#13067=VECTOR('',#60434,1.);
#13068=VECTOR('',#60439,1.);
#13069=VECTOR('',#60442,1.);
#13070=VECTOR('',#60447,1.);
#13071=VECTOR('',#60450,1.);
#13072=VECTOR('',#60455,1.);
#13073=VECTOR('',#60458,1.);
#13074=VECTOR('',#60463,1.);
#13075=VECTOR('',#60466,1.);
#13076=VECTOR('',#60471,1.);
#13077=VECTOR('',#60474,1.);
#13078=VECTOR('',#60479,1.);
#13079=VECTOR('',#60482,1.);
#13080=VECTOR('',#60487,1.);
#13081=VECTOR('',#60490,1.);
#13082=VECTOR('',#60495,1.);
#13083=VECTOR('',#60498,1.);
#13084=VECTOR('',#60503,1.);
#13085=VECTOR('',#60506,1.);
#13086=VECTOR('',#60511,1.);
#13087=VECTOR('',#60514,1.);
#13088=VECTOR('',#60519,1.);
#13089=VECTOR('',#60522,1.);
#13090=VECTOR('',#60527,1.);
#13091=VECTOR('',#60530,1.);
#13092=VECTOR('',#60535,1.);
#13093=VECTOR('',#60538,1.);
#13094=VECTOR('',#60543,1.);
#13095=VECTOR('',#60546,1.);
#13096=VECTOR('',#60551,1.);
#13097=VECTOR('',#60554,1.);
#13098=VECTOR('',#60559,1.);
#13099=VECTOR('',#60562,1.);
#13100=VECTOR('',#60567,1.);
#13101=VECTOR('',#60570,1.);
#13102=VECTOR('',#60575,1.);
#13103=VECTOR('',#60578,1.);
#13104=VECTOR('',#60583,1.);
#13105=VECTOR('',#60586,1.);
#13106=VECTOR('',#60591,1.);
#13107=VECTOR('',#60594,1.);
#13108=VECTOR('',#60599,1.);
#13109=VECTOR('',#60602,1.);
#13110=VECTOR('',#60607,1.);
#13111=VECTOR('',#60610,1.);
#13112=VECTOR('',#60615,1.);
#13113=VECTOR('',#60618,1.);
#13114=VECTOR('',#60623,1.);
#13115=VECTOR('',#60626,1.);
#13116=VECTOR('',#60631,1.);
#13117=VECTOR('',#60634,1.);
#13118=VECTOR('',#60639,1.);
#13119=VECTOR('',#60642,1.);
#13120=VECTOR('',#60647,1.);
#13121=VECTOR('',#60650,1.);
#13122=VECTOR('',#60655,1.);
#13123=VECTOR('',#60658,1.);
#13124=VECTOR('',#60663,1.);
#13125=VECTOR('',#60666,1.);
#13126=VECTOR('',#60671,1.);
#13127=VECTOR('',#60674,1.);
#13128=VECTOR('',#60679,1.);
#13129=VECTOR('',#60682,1.);
#13130=VECTOR('',#60687,1.);
#13131=VECTOR('',#60690,1.);
#13132=VECTOR('',#60695,1.);
#13133=VECTOR('',#60698,1.);
#13134=VECTOR('',#60703,1.);
#13135=VECTOR('',#60704,1.);
#13136=VECTOR('',#60705,1.);
#13137=VECTOR('',#60706,1.);
#13138=VECTOR('',#60707,1.);
#13139=VECTOR('',#60708,1.);
#13140=VECTOR('',#60709,1.);
#13141=VECTOR('',#60710,1.);
#13142=VECTOR('',#60711,1.);
#13143=VECTOR('',#60712,1.);
#13144=VECTOR('',#60713,1.);
#13145=VECTOR('',#60714,1.);
#13146=VECTOR('',#60715,1.);
#13147=VECTOR('',#60716,1.);
#13148=VECTOR('',#60717,1.);
#13149=VECTOR('',#60718,1.);
#13150=VECTOR('',#60719,1.);
#13151=VECTOR('',#60720,1.);
#13152=VECTOR('',#60721,1.);
#13153=VECTOR('',#60722,1.);
#13154=VECTOR('',#60723,1.);
#13155=VECTOR('',#60724,1.);
#13156=VECTOR('',#60725,1.);
#13157=VECTOR('',#60726,1.);
#13158=VECTOR('',#60727,1.);
#13159=VECTOR('',#60728,1.);
#13160=VECTOR('',#60729,1.);
#13161=VECTOR('',#60730,1.);
#13162=VECTOR('',#60731,1.);
#13163=VECTOR('',#60732,1.);
#13164=VECTOR('',#60733,1.);
#13165=VECTOR('',#60734,1.);
#13166=VECTOR('',#60735,1.);
#13167=VECTOR('',#60736,1.);
#13168=VECTOR('',#60737,1.);
#13169=VECTOR('',#60738,1.);
#13170=VECTOR('',#60739,1.);
#13171=VECTOR('',#60740,1.);
#13172=VECTOR('',#60741,1.);
#13173=VECTOR('',#60742,1.);
#13174=VECTOR('',#60743,1.);
#13175=VECTOR('',#60744,1.);
#13176=VECTOR('',#60745,1.);
#13177=VECTOR('',#60746,1.);
#13178=VECTOR('',#60747,1.);
#13179=VECTOR('',#60748,1.);
#13180=VECTOR('',#60749,1.);
#13181=VECTOR('',#60750,1.);
#13182=VECTOR('',#60751,1.);
#13183=VECTOR('',#60752,1.);
#13184=VECTOR('',#60753,1.);
#13185=VECTOR('',#60754,1.);
#13186=VECTOR('',#60755,1.);
#13187=VECTOR('',#60756,1.);
#13188=VECTOR('',#60757,1.);
#13189=VECTOR('',#60758,1.);
#13190=VECTOR('',#60759,1.);
#13191=VECTOR('',#60760,1.);
#13192=VECTOR('',#60761,1.);
#13193=VECTOR('',#60762,1.);
#13194=VECTOR('',#60763,1.);
#13195=VECTOR('',#60764,1.);
#13196=VECTOR('',#60765,1.);
#13197=VECTOR('',#60766,1.);
#13198=VECTOR('',#60767,1.);
#13199=VECTOR('',#60768,1.);
#13200=VECTOR('',#60769,1.);
#13201=VECTOR('',#60770,1.);
#13202=VECTOR('',#60771,1.);
#13203=VECTOR('',#60772,1.);
#13204=VECTOR('',#60773,1.);
#13205=VECTOR('',#60774,1.);
#13206=VECTOR('',#60775,1.);
#13207=VECTOR('',#60776,1.);
#13208=VECTOR('',#60777,1.);
#13209=VECTOR('',#60778,1.);
#13210=VECTOR('',#60779,1.);
#13211=VECTOR('',#60780,1.);
#13212=VECTOR('',#60781,1.);
#13213=VECTOR('',#60782,1.);
#13214=VECTOR('',#60783,1.);
#13215=VECTOR('',#60784,1.);
#13216=VECTOR('',#60785,1.);
#13217=VECTOR('',#60786,1.);
#13218=VECTOR('',#60787,1.);
#13219=VECTOR('',#60788,1.);
#13220=VECTOR('',#60789,1.);
#13221=VECTOR('',#60790,0.999999999999998);
#13222=VECTOR('',#60791,1.);
#13223=VECTOR('',#60792,1.);
#13224=VECTOR('',#60793,1.);
#13225=VECTOR('',#60794,1.);
#13226=VECTOR('',#60795,1.);
#13227=VECTOR('',#60796,1.);
#13228=VECTOR('',#60797,1.);
#13229=VECTOR('',#60798,1.);
#13230=VECTOR('',#60799,1.);
#13231=VECTOR('',#60800,1.);
#13232=VECTOR('',#60801,1.);
#13233=VECTOR('',#60802,1.);
#13234=VECTOR('',#60803,1.);
#13235=VECTOR('',#60804,1.);
#13236=VECTOR('',#60807,1.);
#13237=VECTOR('',#60808,1.);
#13238=VECTOR('',#60809,1.);
#13239=VECTOR('',#60810,1.);
#13240=VECTOR('',#60811,1.);
#13241=VECTOR('',#60812,1.);
#13242=VECTOR('',#60813,1.);
#13243=VECTOR('',#60814,1.);
#13244=VECTOR('',#60815,1.);
#13245=VECTOR('',#60816,1.);
#13246=VECTOR('',#60817,1.);
#13247=VECTOR('',#60818,1.);
#13248=VECTOR('',#60819,1.);
#13249=VECTOR('',#60820,1.);
#13250=VECTOR('',#60821,1.);
#13251=VECTOR('',#60822,1.);
#13252=VECTOR('',#60823,0.999999999999998);
#13253=VECTOR('',#60824,1.);
#13254=VECTOR('',#60825,1.);
#13255=VECTOR('',#60826,1.);
#13256=VECTOR('',#60827,1.);
#13257=VECTOR('',#60828,1.);
#13258=VECTOR('',#60829,1.);
#13259=VECTOR('',#60830,1.);
#13260=VECTOR('',#60831,1.);
#13261=VECTOR('',#60832,1.);
#13262=VECTOR('',#60833,1.);
#13263=VECTOR('',#60834,1.);
#13264=VECTOR('',#60835,1.);
#13265=VECTOR('',#60836,1.);
#13266=VECTOR('',#60837,1.);
#13267=VECTOR('',#60838,1.);
#13268=VECTOR('',#60839,1.);
#13269=VECTOR('',#60840,1.);
#13270=VECTOR('',#60841,1.);
#13271=VECTOR('',#60842,1.);
#13272=VECTOR('',#60843,1.);
#13273=VECTOR('',#60844,1.);
#13274=VECTOR('',#60845,1.);
#13275=VECTOR('',#60846,1.);
#13276=VECTOR('',#60847,1.);
#13277=VECTOR('',#60848,1.);
#13278=VECTOR('',#60849,1.);
#13279=VECTOR('',#60850,1.);
#13280=VECTOR('',#60851,1.);
#13281=VECTOR('',#60852,1.);
#13282=VECTOR('',#60853,1.);
#13283=VECTOR('',#60854,1.);
#13284=VECTOR('',#60855,1.);
#13285=VECTOR('',#60856,1.);
#13286=VECTOR('',#60857,1.);
#13287=VECTOR('',#60858,1.);
#13288=VECTOR('',#60859,1.);
#13289=VECTOR('',#60860,1.);
#13290=VECTOR('',#60861,1.);
#13291=VECTOR('',#60862,1.);
#13292=VECTOR('',#60863,1.);
#13293=VECTOR('',#60864,1.);
#13294=VECTOR('',#60865,1.);
#13295=VECTOR('',#60866,1.);
#13296=VECTOR('',#60867,1.);
#13297=VECTOR('',#60868,1.);
#13298=VECTOR('',#60869,1.);
#13299=VECTOR('',#60870,1.);
#13300=VECTOR('',#60871,1.);
#13301=VECTOR('',#60872,1.);
#13302=VECTOR('',#60873,1.);
#13303=VECTOR('',#60874,1.);
#13304=VECTOR('',#60875,1.);
#13305=VECTOR('',#60876,1.);
#13306=VECTOR('',#60877,1.);
#13307=VECTOR('',#60878,1.);
#13308=VECTOR('',#60879,1.);
#13309=VECTOR('',#60880,1.);
#13310=VECTOR('',#60881,1.);
#13311=VECTOR('',#60882,1.);
#13312=VECTOR('',#60883,1.);
#13313=VECTOR('',#60884,1.);
#13314=VECTOR('',#60885,1.);
#13315=VECTOR('',#60886,1.);
#13316=VECTOR('',#60887,1.);
#13317=VECTOR('',#60888,1.);
#13318=VECTOR('',#60889,1.);
#13319=VECTOR('',#60890,1.);
#13320=VECTOR('',#60891,1.);
#13321=VECTOR('',#60892,1.);
#13322=VECTOR('',#60893,1.);
#13323=VECTOR('',#60894,1.);
#13324=VECTOR('',#60895,1.);
#13325=VECTOR('',#60896,1.);
#13326=VECTOR('',#60897,1.);
#13327=VECTOR('',#60898,1.);
#13328=VECTOR('',#60899,1.);
#13329=VECTOR('',#60900,1.);
#13330=VECTOR('',#60901,1.);
#13331=VECTOR('',#60902,1.);
#13332=VECTOR('',#60903,1.);
#13333=VECTOR('',#60904,1.);
#13334=VECTOR('',#60905,1.);
#13335=VECTOR('',#60906,1.);
#13336=VECTOR('',#60907,1.);
#13337=VECTOR('',#60908,1.);
#13338=VECTOR('',#60919,1.);
#13339=VECTOR('',#60924,1.);
#13340=VECTOR('',#60929,1.);
#13341=VECTOR('',#60934,1.);
#13342=VECTOR('',#60939,1.);
#13343=VECTOR('',#60944,1.);
#13344=VECTOR('',#60949,1.);
#13345=VECTOR('',#60954,1.);
#13346=VECTOR('',#60959,1.);
#13347=VECTOR('',#60964,1.);
#13348=VECTOR('',#60969,1.);
#13349=VECTOR('',#60974,1.);
#13350=VECTOR('',#60979,1.);
#13351=VECTOR('',#60984,1.);
#13352=VECTOR('',#60989,1.);
#13353=VECTOR('',#60994,1.);
#13354=VECTOR('',#60999,1.);
#13355=VECTOR('',#61004,1.);
#13356=VECTOR('',#61009,1.);
#13357=VECTOR('',#61014,1.);
#13358=VECTOR('',#61019,1.);
#13359=VECTOR('',#61024,1.);
#13360=VECTOR('',#61029,1.);
#13361=VECTOR('',#61034,1.);
#13362=VECTOR('',#61039,1.);
#13363=VECTOR('',#61044,1.);
#13364=VECTOR('',#61049,1.);
#13365=VECTOR('',#61054,1.);
#13366=VECTOR('',#61059,1.);
#13367=VECTOR('',#61064,1.);
#13368=VECTOR('',#61069,1.);
#13369=VECTOR('',#61074,1.);
#13370=VECTOR('',#61079,1.);
#13371=VECTOR('',#61084,1.);
#13372=VECTOR('',#61089,1.);
#13373=VECTOR('',#61094,1.);
#13374=VECTOR('',#61099,1.);
#13375=VECTOR('',#61104,1.);
#13376=VECTOR('',#61109,1.);
#13377=VECTOR('',#61114,1.);
#13378=VECTOR('',#61119,1.);
#13379=VECTOR('',#61124,1.);
#13380=VECTOR('',#61129,1.);
#13381=VECTOR('',#61134,1.);
#13382=VECTOR('',#61139,1.);
#13383=VECTOR('',#61144,1.);
#13384=VECTOR('',#61149,1.);
#13385=VECTOR('',#61154,1.);
#13386=VECTOR('',#61159,1.);
#13387=VECTOR('',#61164,1.);
#13388=VECTOR('',#61169,1.);
#16987=CIRCLE('',#49901,0.00400000000001);
#16988=CIRCLE('',#49902,0.00400000000001);
#16989=CIRCLE('',#49904,0.00582500000001);
#16990=CIRCLE('',#49905,0.00582500000001);
#16991=CIRCLE('',#49907,0.01087500000001);
#16992=CIRCLE('',#49908,0.01087500000001);
#16993=CIRCLE('',#49910,0.01087500000001);
#16994=CIRCLE('',#49911,0.01087500000001);
#16995=CIRCLE('',#49913,0.01350000000001);
#16996=CIRCLE('',#49914,0.01350000000001);
#16997=CIRCLE('',#49916,0.01350000000001);
#16998=CIRCLE('',#49917,0.01350000000001);
#16999=CIRCLE('',#49919,0.01350000000001);
#17000=CIRCLE('',#49920,0.01350000000001);
#17001=CIRCLE('',#49922,0.01350000000001);
#17002=CIRCLE('',#49923,0.01350000000001);
#17003=CIRCLE('',#49925,0.01350000000001);
#17004=CIRCLE('',#49926,0.01350000000001);
#17005=CIRCLE('',#49928,0.01350000000001);
#17006=CIRCLE('',#49929,0.01350000000001);
#17007=CIRCLE('',#49931,0.01350000000001);
#17008=CIRCLE('',#49932,0.01350000000001);
#17009=CIRCLE('',#49934,0.01350000000001);
#17010=CIRCLE('',#49935,0.01350000000001);
#17011=CIRCLE('',#49937,0.01350000000001);
#17012=CIRCLE('',#49938,0.01350000000001);
#17013=CIRCLE('',#49940,0.01350000000001);
#17014=CIRCLE('',#49941,0.01350000000001);
#17015=CIRCLE('',#49943,0.01350000000001);
#17016=CIRCLE('',#49944,0.01350000000001);
#17017=CIRCLE('',#49946,0.01350000000001);
#17018=CIRCLE('',#49947,0.01350000000001);
#17019=CIRCLE('',#49949,0.01350000000001);
#17020=CIRCLE('',#49950,0.01350000000001);
#17021=CIRCLE('',#49952,0.01350000000001);
#17022=CIRCLE('',#49953,0.01350000000001);
#17023=CIRCLE('',#49955,0.01350000000001);
#17024=CIRCLE('',#49956,0.01350000000001);
#17025=CIRCLE('',#49958,0.01350000000001);
#17026=CIRCLE('',#49959,0.01350000000001);
#17027=CIRCLE('',#49961,0.01350000000001);
#17028=CIRCLE('',#49962,0.01350000000001);
#17029=CIRCLE('',#49964,0.01350000000001);
#17030=CIRCLE('',#49965,0.01350000000001);
#17031=CIRCLE('',#49967,0.01350000000001);
#17032=CIRCLE('',#49968,0.01350000000001);
#17033=CIRCLE('',#49970,0.01350000000001);
#17034=CIRCLE('',#49971,0.01350000000001);
#17035=CIRCLE('',#49973,0.01350000000001);
#17036=CIRCLE('',#49974,0.01350000000001);
#17037=CIRCLE('',#49976,0.01350000000001);
#17038=CIRCLE('',#49977,0.01350000000001);
#17039=CIRCLE('',#49979,0.01350000000001);
#17040=CIRCLE('',#49980,0.01350000000001);
#17041=CIRCLE('',#49982,0.01350000000001);
#17042=CIRCLE('',#49983,0.01350000000001);
#17043=CIRCLE('',#49985,0.01350000000001);
#17044=CIRCLE('',#49986,0.01350000000001);
#17045=CIRCLE('',#49988,0.01350000000001);
#17046=CIRCLE('',#49989,0.01350000000001);
#17047=CIRCLE('',#49991,0.01350000000001);
#17048=CIRCLE('',#49992,0.01350000000001);
#17049=CIRCLE('',#49994,0.01350000000001);
#17050=CIRCLE('',#49995,0.01350000000001);
#17051=CIRCLE('',#49997,0.01350000000001);
#17052=CIRCLE('',#49998,0.01350000000001);
#17053=CIRCLE('',#50000,0.01350000000001);
#17054=CIRCLE('',#50001,0.01350000000001);
#17055=CIRCLE('',#50003,0.01350000000001);
#17056=CIRCLE('',#50004,0.01350000000001);
#17057=CIRCLE('',#50006,0.01350000000001);
#17058=CIRCLE('',#50007,0.01350000000001);
#17059=CIRCLE('',#50009,0.01350000000001);
#17060=CIRCLE('',#50010,0.01350000000001);
#17061=CIRCLE('',#50012,0.01350000000001);
#17062=CIRCLE('',#50013,0.01350000000001);
#17063=CIRCLE('',#50015,0.01350000000001);
#17064=CIRCLE('',#50016,0.01350000000001);
#17065=CIRCLE('',#50018,0.01350000000001);
#17066=CIRCLE('',#50019,0.01350000000001);
#17067=CIRCLE('',#50021,0.01350000000001);
#17068=CIRCLE('',#50022,0.01350000000001);
#17069=CIRCLE('',#50024,0.01350000000001);
#17070=CIRCLE('',#50025,0.01350000000001);
#17071=CIRCLE('',#50027,0.01350000000001);
#17072=CIRCLE('',#50028,0.01350000000001);
#17073=CIRCLE('',#50030,0.01350000000001);
#17074=CIRCLE('',#50031,0.01350000000001);
#17075=CIRCLE('',#50033,0.01350000000001);
#17076=CIRCLE('',#50034,0.01350000000001);
#17077=CIRCLE('',#50036,0.01350000000001);
#17078=CIRCLE('',#50037,0.01350000000001);
#17079=CIRCLE('',#50039,0.01350000000001);
#17080=CIRCLE('',#50040,0.01350000000001);
#17081=CIRCLE('',#50042,0.01350000000001);
#17082=CIRCLE('',#50043,0.01350000000001);
#17083=CIRCLE('',#50045,0.01350000000001);
#17084=CIRCLE('',#50046,0.01350000000001);
#17085=CIRCLE('',#50048,0.01350000000001);
#17086=CIRCLE('',#50049,0.01350000000001);
#17087=CIRCLE('',#50051,0.01350000000001);
#17088=CIRCLE('',#50052,0.01350000000001);
#17089=CIRCLE('',#50054,0.01350000000001);
#17090=CIRCLE('',#50055,0.01350000000001);
#17091=CIRCLE('',#50057,0.01350000000001);
#17092=CIRCLE('',#50058,0.01350000000001);
#17093=CIRCLE('',#50060,0.01350000000001);
#17094=CIRCLE('',#50061,0.01350000000001);
#17095=CIRCLE('',#50063,0.01350000000001);
#17096=CIRCLE('',#50064,0.01350000000001);
#20691=VERTEX_POINT('',#106263);
#20692=VERTEX_POINT('',#106265);
#20693=VERTEX_POINT('',#106269);
#20694=VERTEX_POINT('',#106271);
#20695=VERTEX_POINT('',#106275);
#20696=VERTEX_POINT('',#106277);
#20697=VERTEX_POINT('',#106281);
#20698=VERTEX_POINT('',#106283);
#20699=VERTEX_POINT('',#106287);
#20700=VERTEX_POINT('',#106288);
#20701=VERTEX_POINT('',#106290);
#20702=VERTEX_POINT('',#106292);
#20703=VERTEX_POINT('',#106296);
#20704=VERTEX_POINT('',#106297);
#20705=VERTEX_POINT('',#106299);
#20706=VERTEX_POINT('',#106301);
#20707=VERTEX_POINT('',#106305);
#20708=VERTEX_POINT('',#106306);
#20709=VERTEX_POINT('',#106308);
#20710=VERTEX_POINT('',#106310);
#20711=VERTEX_POINT('',#106314);
#20712=VERTEX_POINT('',#106315);
#20713=VERTEX_POINT('',#106317);
#20714=VERTEX_POINT('',#106319);
#20715=VERTEX_POINT('',#106323);
#20716=VERTEX_POINT('',#106324);
#20717=VERTEX_POINT('',#106326);
#20718=VERTEX_POINT('',#106328);
#20719=VERTEX_POINT('',#106332);
#20720=VERTEX_POINT('',#106333);
#20721=VERTEX_POINT('',#106335);
#20722=VERTEX_POINT('',#106337);
#20723=VERTEX_POINT('',#106341);
#20724=VERTEX_POINT('',#106342);
#20725=VERTEX_POINT('',#106344);
#20726=VERTEX_POINT('',#106346);
#20727=VERTEX_POINT('',#106350);
#20728=VERTEX_POINT('',#106351);
#20729=VERTEX_POINT('',#106353);
#20730=VERTEX_POINT('',#106355);
#20731=VERTEX_POINT('',#106359);
#20732=VERTEX_POINT('',#106360);
#20733=VERTEX_POINT('',#106362);
#20734=VERTEX_POINT('',#106364);
#20735=VERTEX_POINT('',#106368);
#20736=VERTEX_POINT('',#106369);
#20737=VERTEX_POINT('',#106371);
#20738=VERTEX_POINT('',#106373);
#20739=VERTEX_POINT('',#106377);
#20740=VERTEX_POINT('',#106378);
#20741=VERTEX_POINT('',#106380);
#20742=VERTEX_POINT('',#106382);
#20743=VERTEX_POINT('',#106386);
#20744=VERTEX_POINT('',#106387);
#20745=VERTEX_POINT('',#106389);
#20746=VERTEX_POINT('',#106391);
#20747=VERTEX_POINT('',#106395);
#20748=VERTEX_POINT('',#106396);
#20749=VERTEX_POINT('',#106398);
#20750=VERTEX_POINT('',#106400);
#20751=VERTEX_POINT('',#106404);
#20752=VERTEX_POINT('',#106405);
#20753=VERTEX_POINT('',#106407);
#20754=VERTEX_POINT('',#106409);
#20755=VERTEX_POINT('',#106413);
#20756=VERTEX_POINT('',#106414);
#20757=VERTEX_POINT('',#106416);
#20758=VERTEX_POINT('',#106418);
#20759=VERTEX_POINT('',#106422);
#20760=VERTEX_POINT('',#106423);
#20761=VERTEX_POINT('',#106425);
#20762=VERTEX_POINT('',#106427);
#20763=VERTEX_POINT('',#106431);
#20764=VERTEX_POINT('',#106432);
#20765=VERTEX_POINT('',#106434);
#20766=VERTEX_POINT('',#106436);
#20767=VERTEX_POINT('',#106440);
#20768=VERTEX_POINT('',#106441);
#20769=VERTEX_POINT('',#106443);
#20770=VERTEX_POINT('',#106445);
#20771=VERTEX_POINT('',#106449);
#20772=VERTEX_POINT('',#106450);
#20773=VERTEX_POINT('',#106452);
#20774=VERTEX_POINT('',#106454);
#20775=VERTEX_POINT('',#106458);
#20776=VERTEX_POINT('',#106459);
#20777=VERTEX_POINT('',#106461);
#20778=VERTEX_POINT('',#106463);
#20779=VERTEX_POINT('',#106467);
#20780=VERTEX_POINT('',#106468);
#20781=VERTEX_POINT('',#106470);
#20782=VERTEX_POINT('',#106472);
#20783=VERTEX_POINT('',#106476);
#20784=VERTEX_POINT('',#106477);
#20785=VERTEX_POINT('',#106479);
#20786=VERTEX_POINT('',#106481);
#20787=VERTEX_POINT('',#106485);
#20788=VERTEX_POINT('',#106486);
#20789=VERTEX_POINT('',#106488);
#20790=VERTEX_POINT('',#106490);
#20791=VERTEX_POINT('',#106494);
#20792=VERTEX_POINT('',#106495);
#20793=VERTEX_POINT('',#106497);
#20794=VERTEX_POINT('',#106499);
#20795=VERTEX_POINT('',#106503);
#20796=VERTEX_POINT('',#106504);
#20797=VERTEX_POINT('',#106506);
#20798=VERTEX_POINT('',#106508);
#20799=VERTEX_POINT('',#106512);
#20800=VERTEX_POINT('',#106513);
#20801=VERTEX_POINT('',#106515);
#20802=VERTEX_POINT('',#106517);
#20803=VERTEX_POINT('',#106521);
#20804=VERTEX_POINT('',#106522);
#20805=VERTEX_POINT('',#106524);
#20806=VERTEX_POINT('',#106526);
#20807=VERTEX_POINT('',#106530);
#20808=VERTEX_POINT('',#106531);
#20809=VERTEX_POINT('',#106533);
#20810=VERTEX_POINT('',#106535);
#20811=VERTEX_POINT('',#106539);
#20812=VERTEX_POINT('',#106540);
#20813=VERTEX_POINT('',#106542);
#20814=VERTEX_POINT('',#106544);
#20815=VERTEX_POINT('',#106548);
#20816=VERTEX_POINT('',#106549);
#20817=VERTEX_POINT('',#106551);
#20818=VERTEX_POINT('',#106553);
#20819=VERTEX_POINT('',#106557);
#20820=VERTEX_POINT('',#106558);
#20821=VERTEX_POINT('',#106560);
#20822=VERTEX_POINT('',#106562);
#20823=VERTEX_POINT('',#106566);
#20824=VERTEX_POINT('',#106567);
#20825=VERTEX_POINT('',#106569);
#20826=VERTEX_POINT('',#106571);
#20827=VERTEX_POINT('',#106575);
#20828=VERTEX_POINT('',#106576);
#20829=VERTEX_POINT('',#106578);
#20830=VERTEX_POINT('',#106580);
#20831=VERTEX_POINT('',#106584);
#20832=VERTEX_POINT('',#106585);
#20833=VERTEX_POINT('',#106587);
#20834=VERTEX_POINT('',#106589);
#20835=VERTEX_POINT('',#106593);
#20836=VERTEX_POINT('',#106594);
#20837=VERTEX_POINT('',#106596);
#20838=VERTEX_POINT('',#106598);
#20839=VERTEX_POINT('',#106602);
#20840=VERTEX_POINT('',#106603);
#20841=VERTEX_POINT('',#106605);
#20842=VERTEX_POINT('',#106607);
#20843=VERTEX_POINT('',#106611);
#20844=VERTEX_POINT('',#106612);
#20845=VERTEX_POINT('',#106614);
#20846=VERTEX_POINT('',#106616);
#20847=VERTEX_POINT('',#106620);
#20848=VERTEX_POINT('',#106621);
#20849=VERTEX_POINT('',#106623);
#20850=VERTEX_POINT('',#106625);
#20851=VERTEX_POINT('',#106629);
#20852=VERTEX_POINT('',#106630);
#20853=VERTEX_POINT('',#106632);
#20854=VERTEX_POINT('',#106634);
#20855=VERTEX_POINT('',#106638);
#20856=VERTEX_POINT('',#106639);
#20857=VERTEX_POINT('',#106641);
#20858=VERTEX_POINT('',#106643);
#20859=VERTEX_POINT('',#106647);
#20860=VERTEX_POINT('',#106648);
#20861=VERTEX_POINT('',#106650);
#20862=VERTEX_POINT('',#106652);
#20863=VERTEX_POINT('',#106656);
#20864=VERTEX_POINT('',#106657);
#20865=VERTEX_POINT('',#106659);
#20866=VERTEX_POINT('',#106661);
#20867=VERTEX_POINT('',#106665);
#20868=VERTEX_POINT('',#106666);
#20869=VERTEX_POINT('',#106668);
#20870=VERTEX_POINT('',#106670);
#20871=VERTEX_POINT('',#106674);
#20872=VERTEX_POINT('',#106675);
#20873=VERTEX_POINT('',#106677);
#20874=VERTEX_POINT('',#106679);
#20875=VERTEX_POINT('',#106683);
#20876=VERTEX_POINT('',#106684);
#20877=VERTEX_POINT('',#106686);
#20878=VERTEX_POINT('',#106688);
#20879=VERTEX_POINT('',#106692);
#20880=VERTEX_POINT('',#106693);
#20881=VERTEX_POINT('',#106695);
#20882=VERTEX_POINT('',#106697);
#20883=VERTEX_POINT('',#106701);
#20884=VERTEX_POINT('',#106702);
#20885=VERTEX_POINT('',#106704);
#20886=VERTEX_POINT('',#106706);
#20887=VERTEX_POINT('',#106710);
#20888=VERTEX_POINT('',#106711);
#20889=VERTEX_POINT('',#106713);
#20890=VERTEX_POINT('',#106715);
#20891=VERTEX_POINT('',#106719);
#20892=VERTEX_POINT('',#106720);
#20893=VERTEX_POINT('',#106722);
#20894=VERTEX_POINT('',#106724);
#20895=VERTEX_POINT('',#106728);
#20896=VERTEX_POINT('',#106729);
#20897=VERTEX_POINT('',#106731);
#20898=VERTEX_POINT('',#106733);
#20899=VERTEX_POINT('',#106737);
#20900=VERTEX_POINT('',#106738);
#20901=VERTEX_POINT('',#106740);
#20902=VERTEX_POINT('',#106742);
#20903=VERTEX_POINT('',#106746);
#20904=VERTEX_POINT('',#106749);
#20905=VERTEX_POINT('',#106752);
#20906=VERTEX_POINT('',#106755);
#20907=VERTEX_POINT('',#106758);
#20908=VERTEX_POINT('',#106761);
#20909=VERTEX_POINT('',#106764);
#20910=VERTEX_POINT('',#106767);
#20911=VERTEX_POINT('',#106770);
#20912=VERTEX_POINT('',#106773);
#20913=VERTEX_POINT('',#106776);
#20914=VERTEX_POINT('',#106779);
#20915=VERTEX_POINT('',#106782);
#20916=VERTEX_POINT('',#106785);
#20917=VERTEX_POINT('',#106788);
#20918=VERTEX_POINT('',#106791);
#20919=VERTEX_POINT('',#106794);
#20920=VERTEX_POINT('',#106797);
#20921=VERTEX_POINT('',#106800);
#20922=VERTEX_POINT('',#106803);
#20923=VERTEX_POINT('',#106806);
#20924=VERTEX_POINT('',#106809);
#20925=VERTEX_POINT('',#106812);
#20926=VERTEX_POINT('',#106815);
#20927=VERTEX_POINT('',#106818);
#20928=VERTEX_POINT('',#106821);
#20929=VERTEX_POINT('',#106824);
#20930=VERTEX_POINT('',#106827);
#20931=VERTEX_POINT('',#106830);
#20932=VERTEX_POINT('',#106833);
#20933=VERTEX_POINT('',#106836);
#20934=VERTEX_POINT('',#106839);
#20935=VERTEX_POINT('',#106842);
#20936=VERTEX_POINT('',#106845);
#20937=VERTEX_POINT('',#106848);
#20938=VERTEX_POINT('',#106851);
#20939=VERTEX_POINT('',#106854);
#20940=VERTEX_POINT('',#106857);
#20941=VERTEX_POINT('',#106860);
#20942=VERTEX_POINT('',#106863);
#20943=VERTEX_POINT('',#106866);
#20944=VERTEX_POINT('',#106869);
#20945=VERTEX_POINT('',#106872);
#20946=VERTEX_POINT('',#106875);
#20947=VERTEX_POINT('',#106878);
#20948=VERTEX_POINT('',#106881);
#20949=VERTEX_POINT('',#106884);
#20950=VERTEX_POINT('',#106887);
#20951=VERTEX_POINT('',#106890);
#20952=VERTEX_POINT('',#106893);
#20953=VERTEX_POINT('',#106896);
#20954=VERTEX_POINT('',#106900);
#20955=VERTEX_POINT('',#106903);
#20956=VERTEX_POINT('',#106906);
#20957=VERTEX_POINT('',#106909);
#20958=VERTEX_POINT('',#106912);
#20959=VERTEX_POINT('',#106915);
#20960=VERTEX_POINT('',#106918);
#20961=VERTEX_POINT('',#106921);
#20962=VERTEX_POINT('',#106924);
#20963=VERTEX_POINT('',#106927);
#20964=VERTEX_POINT('',#106930);
#20965=VERTEX_POINT('',#106933);
#20966=VERTEX_POINT('',#106936);
#20967=VERTEX_POINT('',#106939);
#20968=VERTEX_POINT('',#106942);
#20969=VERTEX_POINT('',#106945);
#20970=VERTEX_POINT('',#106948);
#20971=VERTEX_POINT('',#106951);
#20972=VERTEX_POINT('',#106954);
#20973=VERTEX_POINT('',#106957);
#20974=VERTEX_POINT('',#106960);
#20975=VERTEX_POINT('',#106963);
#20976=VERTEX_POINT('',#106966);
#20977=VERTEX_POINT('',#106969);
#20978=VERTEX_POINT('',#106972);
#20979=VERTEX_POINT('',#106975);
#20980=VERTEX_POINT('',#106978);
#20981=VERTEX_POINT('',#106981);
#20982=VERTEX_POINT('',#106984);
#20983=VERTEX_POINT('',#106987);
#20984=VERTEX_POINT('',#106990);
#20985=VERTEX_POINT('',#106993);
#20986=VERTEX_POINT('',#106996);
#20987=VERTEX_POINT('',#106999);
#20988=VERTEX_POINT('',#107002);
#20989=VERTEX_POINT('',#107005);
#20990=VERTEX_POINT('',#107008);
#20991=VERTEX_POINT('',#107011);
#20992=VERTEX_POINT('',#107014);
#20993=VERTEX_POINT('',#107017);
#20994=VERTEX_POINT('',#107020);
#20995=VERTEX_POINT('',#107023);
#20996=VERTEX_POINT('',#107026);
#20997=VERTEX_POINT('',#107029);
#20998=VERTEX_POINT('',#107032);
#20999=VERTEX_POINT('',#107035);
#21000=VERTEX_POINT('',#107038);
#21001=VERTEX_POINT('',#107041);
#21002=VERTEX_POINT('',#107044);
#21003=VERTEX_POINT('',#107047);
#21004=VERTEX_POINT('',#107050);
#27348=EDGE_CURVE('',#20691,#20691,#16987,.T.);
#27349=EDGE_CURVE('',#20691,#20692,#11044,.T.);
#27350=EDGE_CURVE('',#20692,#20692,#16988,.T.);
#27351=EDGE_CURVE('',#20693,#20693,#16989,.T.);
#27352=EDGE_CURVE('',#20693,#20694,#11045,.T.);
#27353=EDGE_CURVE('',#20694,#20694,#16990,.T.);
#27354=EDGE_CURVE('',#20695,#20695,#16991,.T.);
#27355=EDGE_CURVE('',#20695,#20696,#11046,.T.);
#27356=EDGE_CURVE('',#20696,#20696,#16992,.T.);
#27357=EDGE_CURVE('',#20697,#20697,#16993,.T.);
#27358=EDGE_CURVE('',#20697,#20698,#11047,.T.);
#27359=EDGE_CURVE('',#20698,#20698,#16994,.T.);
#27360=EDGE_CURVE('',#20699,#20700,#11048,.T.);
#27361=EDGE_CURVE('',#20701,#20700,#16995,.T.);
#27362=EDGE_CURVE('',#20702,#20701,#11049,.T.);
#27363=EDGE_CURVE('',#20702,#20699,#16996,.T.);
#27364=EDGE_CURVE('',#20703,#20704,#11050,.T.);
#27365=EDGE_CURVE('',#20703,#20705,#16997,.T.);
#27366=EDGE_CURVE('',#20705,#20706,#11051,.T.);
#27367=EDGE_CURVE('',#20704,#20706,#16998,.T.);
#27368=EDGE_CURVE('',#20707,#20708,#11052,.T.);
#27369=EDGE_CURVE('',#20707,#20709,#16999,.T.);
#27370=EDGE_CURVE('',#20709,#20710,#11053,.T.);
#27371=EDGE_CURVE('',#20708,#20710,#17000,.T.);
#27372=EDGE_CURVE('',#20711,#20712,#11054,.T.);
#27373=EDGE_CURVE('',#20711,#20713,#17001,.T.);
#27374=EDGE_CURVE('',#20713,#20714,#11055,.T.);
#27375=EDGE_CURVE('',#20712,#20714,#17002,.T.);
#27376=EDGE_CURVE('',#20715,#20716,#11056,.T.);
#27377=EDGE_CURVE('',#20715,#20717,#17003,.T.);
#27378=EDGE_CURVE('',#20717,#20718,#11057,.T.);
#27379=EDGE_CURVE('',#20716,#20718,#17004,.T.);
#27380=EDGE_CURVE('',#20719,#20720,#11058,.T.);
#27381=EDGE_CURVE('',#20719,#20721,#17005,.T.);
#27382=EDGE_CURVE('',#20721,#20722,#11059,.T.);
#27383=EDGE_CURVE('',#20720,#20722,#17006,.T.);
#27384=EDGE_CURVE('',#20723,#20724,#11060,.T.);
#27385=EDGE_CURVE('',#20723,#20725,#17007,.T.);
#27386=EDGE_CURVE('',#20725,#20726,#11061,.T.);
#27387=EDGE_CURVE('',#20724,#20726,#17008,.T.);
#27388=EDGE_CURVE('',#20727,#20728,#11062,.T.);
#27389=EDGE_CURVE('',#20727,#20729,#17009,.T.);
#27390=EDGE_CURVE('',#20729,#20730,#11063,.T.);
#27391=EDGE_CURVE('',#20728,#20730,#17010,.T.);
#27392=EDGE_CURVE('',#20731,#20732,#11064,.T.);
#27393=EDGE_CURVE('',#20731,#20733,#17011,.T.);
#27394=EDGE_CURVE('',#20733,#20734,#11065,.T.);
#27395=EDGE_CURVE('',#20732,#20734,#17012,.T.);
#27396=EDGE_CURVE('',#20735,#20736,#11066,.T.);
#27397=EDGE_CURVE('',#20735,#20737,#17013,.T.);
#27398=EDGE_CURVE('',#20737,#20738,#11067,.T.);
#27399=EDGE_CURVE('',#20736,#20738,#17014,.T.);
#27400=EDGE_CURVE('',#20739,#20740,#11068,.T.);
#27401=EDGE_CURVE('',#20739,#20741,#17015,.T.);
#27402=EDGE_CURVE('',#20741,#20742,#11069,.T.);
#27403=EDGE_CURVE('',#20740,#20742,#17016,.T.);
#27404=EDGE_CURVE('',#20743,#20744,#11070,.T.);
#27405=EDGE_CURVE('',#20743,#20745,#17017,.T.);
#27406=EDGE_CURVE('',#20745,#20746,#11071,.T.);
#27407=EDGE_CURVE('',#20744,#20746,#17018,.T.);
#27408=EDGE_CURVE('',#20747,#20748,#11072,.T.);
#27409=EDGE_CURVE('',#20747,#20749,#17019,.T.);
#27410=EDGE_CURVE('',#20749,#20750,#11073,.T.);
#27411=EDGE_CURVE('',#20748,#20750,#17020,.T.);
#27412=EDGE_CURVE('',#20751,#20752,#11074,.T.);
#27413=EDGE_CURVE('',#20751,#20753,#17021,.T.);
#27414=EDGE_CURVE('',#20753,#20754,#11075,.T.);
#27415=EDGE_CURVE('',#20752,#20754,#17022,.T.);
#27416=EDGE_CURVE('',#20755,#20756,#11076,.T.);
#27417=EDGE_CURVE('',#20755,#20757,#17023,.T.);
#27418=EDGE_CURVE('',#20757,#20758,#11077,.T.);
#27419=EDGE_CURVE('',#20756,#20758,#17024,.T.);
#27420=EDGE_CURVE('',#20759,#20760,#11078,.T.);
#27421=EDGE_CURVE('',#20759,#20761,#17025,.T.);
#27422=EDGE_CURVE('',#20761,#20762,#11079,.T.);
#27423=EDGE_CURVE('',#20760,#20762,#17026,.T.);
#27424=EDGE_CURVE('',#20763,#20764,#11080,.T.);
#27425=EDGE_CURVE('',#20765,#20764,#17027,.T.);
#27426=EDGE_CURVE('',#20766,#20765,#11081,.T.);
#27427=EDGE_CURVE('',#20766,#20763,#17028,.T.);
#27428=EDGE_CURVE('',#20767,#20768,#11082,.T.);
#27429=EDGE_CURVE('',#20769,#20768,#17029,.T.);
#27430=EDGE_CURVE('',#20770,#20769,#11083,.T.);
#27431=EDGE_CURVE('',#20770,#20767,#17030,.T.);
#27432=EDGE_CURVE('',#20771,#20772,#11084,.T.);
#27433=EDGE_CURVE('',#20773,#20772,#17031,.T.);
#27434=EDGE_CURVE('',#20774,#20773,#11085,.T.);
#27435=EDGE_CURVE('',#20774,#20771,#17032,.T.);
#27436=EDGE_CURVE('',#20775,#20776,#11086,.T.);
#27437=EDGE_CURVE('',#20775,#20777,#17033,.T.);
#27438=EDGE_CURVE('',#20777,#20778,#11087,.T.);
#27439=EDGE_CURVE('',#20776,#20778,#17034,.T.);
#27440=EDGE_CURVE('',#20779,#20780,#11088,.T.);
#27441=EDGE_CURVE('',#20779,#20781,#17035,.T.);
#27442=EDGE_CURVE('',#20781,#20782,#11089,.T.);
#27443=EDGE_CURVE('',#20780,#20782,#17036,.T.);
#27444=EDGE_CURVE('',#20783,#20784,#11090,.T.);
#27445=EDGE_CURVE('',#20783,#20785,#17037,.T.);
#27446=EDGE_CURVE('',#20785,#20786,#11091,.T.);
#27447=EDGE_CURVE('',#20784,#20786,#17038,.T.);
#27448=EDGE_CURVE('',#20787,#20788,#11092,.T.);
#27449=EDGE_CURVE('',#20787,#20789,#17039,.T.);
#27450=EDGE_CURVE('',#20789,#20790,#11093,.T.);
#27451=EDGE_CURVE('',#20788,#20790,#17040,.T.);
#27452=EDGE_CURVE('',#20791,#20792,#11094,.T.);
#27453=EDGE_CURVE('',#20791,#20793,#17041,.T.);
#27454=EDGE_CURVE('',#20793,#20794,#11095,.T.);
#27455=EDGE_CURVE('',#20792,#20794,#17042,.T.);
#27456=EDGE_CURVE('',#20795,#20796,#11096,.T.);
#27457=EDGE_CURVE('',#20795,#20797,#17043,.T.);
#27458=EDGE_CURVE('',#20797,#20798,#11097,.T.);
#27459=EDGE_CURVE('',#20796,#20798,#17044,.T.);
#27460=EDGE_CURVE('',#20799,#20800,#11098,.T.);
#27461=EDGE_CURVE('',#20799,#20801,#17045,.T.);
#27462=EDGE_CURVE('',#20801,#20802,#11099,.T.);
#27463=EDGE_CURVE('',#20800,#20802,#17046,.T.);
#27464=EDGE_CURVE('',#20803,#20804,#11100,.T.);
#27465=EDGE_CURVE('',#20803,#20805,#17047,.T.);
#27466=EDGE_CURVE('',#20805,#20806,#11101,.T.);
#27467=EDGE_CURVE('',#20804,#20806,#17048,.T.);
#27468=EDGE_CURVE('',#20807,#20808,#11102,.T.);
#27469=EDGE_CURVE('',#20807,#20809,#17049,.T.);
#27470=EDGE_CURVE('',#20809,#20810,#11103,.T.);
#27471=EDGE_CURVE('',#20808,#20810,#17050,.T.);
#27472=EDGE_CURVE('',#20811,#20812,#11104,.T.);
#27473=EDGE_CURVE('',#20811,#20813,#17051,.T.);
#27474=EDGE_CURVE('',#20813,#20814,#11105,.T.);
#27475=EDGE_CURVE('',#20812,#20814,#17052,.T.);
#27476=EDGE_CURVE('',#20815,#20816,#11106,.T.);
#27477=EDGE_CURVE('',#20815,#20817,#17053,.T.);
#27478=EDGE_CURVE('',#20817,#20818,#11107,.T.);
#27479=EDGE_CURVE('',#20816,#20818,#17054,.T.);
#27480=EDGE_CURVE('',#20819,#20820,#11108,.T.);
#27481=EDGE_CURVE('',#20821,#20820,#17055,.T.);
#27482=EDGE_CURVE('',#20822,#20821,#11109,.T.);
#27483=EDGE_CURVE('',#20822,#20819,#17056,.T.);
#27484=EDGE_CURVE('',#20823,#20824,#11110,.T.);
#27485=EDGE_CURVE('',#20823,#20825,#17057,.T.);
#27486=EDGE_CURVE('',#20825,#20826,#11111,.T.);
#27487=EDGE_CURVE('',#20824,#20826,#17058,.T.);
#27488=EDGE_CURVE('',#20827,#20828,#11112,.T.);
#27489=EDGE_CURVE('',#20827,#20829,#17059,.T.);
#27490=EDGE_CURVE('',#20829,#20830,#11113,.T.);
#27491=EDGE_CURVE('',#20828,#20830,#17060,.T.);
#27492=EDGE_CURVE('',#20831,#20832,#11114,.T.);
#27493=EDGE_CURVE('',#20831,#20833,#17061,.T.);
#27494=EDGE_CURVE('',#20833,#20834,#11115,.T.);
#27495=EDGE_CURVE('',#20832,#20834,#17062,.T.);
#27496=EDGE_CURVE('',#20835,#20836,#11116,.T.);
#27497=EDGE_CURVE('',#20835,#20837,#17063,.T.);
#27498=EDGE_CURVE('',#20837,#20838,#11117,.T.);
#27499=EDGE_CURVE('',#20836,#20838,#17064,.T.);
#27500=EDGE_CURVE('',#20839,#20840,#11118,.T.);
#27501=EDGE_CURVE('',#20839,#20841,#17065,.T.);
#27502=EDGE_CURVE('',#20841,#20842,#11119,.T.);
#27503=EDGE_CURVE('',#20840,#20842,#17066,.T.);
#27504=EDGE_CURVE('',#20843,#20844,#11120,.T.);
#27505=EDGE_CURVE('',#20843,#20845,#17067,.T.);
#27506=EDGE_CURVE('',#20845,#20846,#11121,.T.);
#27507=EDGE_CURVE('',#20844,#20846,#17068,.T.);
#27508=EDGE_CURVE('',#20847,#20848,#11122,.T.);
#27509=EDGE_CURVE('',#20847,#20849,#17069,.T.);
#27510=EDGE_CURVE('',#20849,#20850,#11123,.T.);
#27511=EDGE_CURVE('',#20848,#20850,#17070,.T.);
#27512=EDGE_CURVE('',#20851,#20852,#11124,.T.);
#27513=EDGE_CURVE('',#20851,#20853,#17071,.T.);
#27514=EDGE_CURVE('',#20853,#20854,#11125,.T.);
#27515=EDGE_CURVE('',#20852,#20854,#17072,.T.);
#27516=EDGE_CURVE('',#20855,#20856,#11126,.T.);
#27517=EDGE_CURVE('',#20855,#20857,#17073,.T.);
#27518=EDGE_CURVE('',#20857,#20858,#11127,.T.);
#27519=EDGE_CURVE('',#20856,#20858,#17074,.T.);
#27520=EDGE_CURVE('',#20859,#20860,#11128,.T.);
#27521=EDGE_CURVE('',#20861,#20860,#17075,.T.);
#27522=EDGE_CURVE('',#20862,#20861,#11129,.T.);
#27523=EDGE_CURVE('',#20862,#20859,#17076,.T.);
#27524=EDGE_CURVE('',#20863,#20864,#11130,.T.);
#27525=EDGE_CURVE('',#20865,#20864,#17077,.T.);
#27526=EDGE_CURVE('',#20866,#20865,#11131,.T.);
#27527=EDGE_CURVE('',#20866,#20863,#17078,.T.);
#27528=EDGE_CURVE('',#20867,#20868,#11132,.T.);
#27529=EDGE_CURVE('',#20869,#20868,#17079,.T.);
#27530=EDGE_CURVE('',#20870,#20869,#11133,.T.);
#27531=EDGE_CURVE('',#20870,#20867,#17080,.T.);
#27532=EDGE_CURVE('',#20871,#20872,#11134,.T.);
#27533=EDGE_CURVE('',#20873,#20872,#17081,.T.);
#27534=EDGE_CURVE('',#20874,#20873,#11135,.T.);
#27535=EDGE_CURVE('',#20874,#20871,#17082,.T.);
#27536=EDGE_CURVE('',#20875,#20876,#11136,.T.);
#27537=EDGE_CURVE('',#20877,#20876,#17083,.T.);
#27538=EDGE_CURVE('',#20878,#20877,#11137,.T.);
#27539=EDGE_CURVE('',#20878,#20875,#17084,.T.);
#27540=EDGE_CURVE('',#20879,#20880,#11138,.T.);
#27541=EDGE_CURVE('',#20881,#20880,#17085,.T.);
#27542=EDGE_CURVE('',#20882,#20881,#11139,.T.);
#27543=EDGE_CURVE('',#20882,#20879,#17086,.T.);
#27544=EDGE_CURVE('',#20883,#20884,#11140,.T.);
#27545=EDGE_CURVE('',#20885,#20884,#17087,.T.);
#27546=EDGE_CURVE('',#20886,#20885,#11141,.T.);
#27547=EDGE_CURVE('',#20886,#20883,#17088,.T.);
#27548=EDGE_CURVE('',#20887,#20888,#11142,.T.);
#27549=EDGE_CURVE('',#20887,#20889,#17089,.T.);
#27550=EDGE_CURVE('',#20889,#20890,#11143,.T.);
#27551=EDGE_CURVE('',#20888,#20890,#17090,.T.);
#27552=EDGE_CURVE('',#20891,#20892,#11144,.T.);
#27553=EDGE_CURVE('',#20891,#20893,#17091,.T.);
#27554=EDGE_CURVE('',#20893,#20894,#11145,.T.);
#27555=EDGE_CURVE('',#20892,#20894,#17092,.T.);
#27556=EDGE_CURVE('',#20895,#20896,#11146,.T.);
#27557=EDGE_CURVE('',#20897,#20896,#17093,.T.);
#27558=EDGE_CURVE('',#20898,#20897,#11147,.T.);
#27559=EDGE_CURVE('',#20898,#20895,#17094,.T.);
#27560=EDGE_CURVE('',#20899,#20900,#11148,.T.);
#27561=EDGE_CURVE('',#20899,#20901,#17095,.T.);
#27562=EDGE_CURVE('',#20901,#20902,#11149,.T.);
#27563=EDGE_CURVE('',#20900,#20902,#17096,.T.);
#27564=EDGE_CURVE('',#20903,#20703,#11150,.T.);
#27565=EDGE_CURVE('',#20699,#20903,#11151,.T.);
#27566=EDGE_CURVE('',#20904,#20702,#11152,.T.);
#27567=EDGE_CURVE('',#20895,#20904,#11153,.T.);
#27568=EDGE_CURVE('',#20905,#20898,#11154,.T.);
#27569=EDGE_CURVE('',#20901,#20905,#11155,.T.);
#27570=EDGE_CURVE('',#20906,#20899,#11156,.T.);
#27571=EDGE_CURVE('',#20893,#20906,#11157,.T.);
#27572=EDGE_CURVE('',#20907,#20891,#11158,.T.);
#27573=EDGE_CURVE('',#20859,#20907,#11159,.T.);
#27574=EDGE_CURVE('',#20908,#20862,#11160,.T.);
#27575=EDGE_CURVE('',#20863,#20908,#11161,.T.);
#27576=EDGE_CURVE('',#20909,#20866,#11162,.T.);
#27577=EDGE_CURVE('',#20867,#20909,#11163,.T.);
#27578=EDGE_CURVE('',#20910,#20870,#11164,.T.);
#27579=EDGE_CURVE('',#20871,#20910,#11165,.T.);
#27580=EDGE_CURVE('',#20911,#20874,#11166,.T.);
#27581=EDGE_CURVE('',#20875,#20911,#11167,.T.);
#27582=EDGE_CURVE('',#20912,#20878,#11168,.T.);
#27583=EDGE_CURVE('',#20879,#20912,#11169,.T.);
#27584=EDGE_CURVE('',#20913,#20882,#11170,.T.);
#27585=EDGE_CURVE('',#20883,#20913,#11171,.T.);
#27586=EDGE_CURVE('',#20914,#20886,#11172,.T.);
#27587=EDGE_CURVE('',#20889,#20914,#11173,.T.);
#27588=EDGE_CURVE('',#20915,#20887,#11174,.T.);
#27589=EDGE_CURVE('',#20857,#20915,#11175,.T.);
#27590=EDGE_CURVE('',#20916,#20855,#11176,.T.);
#27591=EDGE_CURVE('',#20853,#20916,#11177,.T.);
#27592=EDGE_CURVE('',#20917,#20851,#11178,.T.);
#27593=EDGE_CURVE('',#20849,#20917,#11179,.T.);
#27594=EDGE_CURVE('',#20918,#20847,#11180,.T.);
#27595=EDGE_CURVE('',#20845,#20918,#11181,.T.);
#27596=EDGE_CURVE('',#20919,#20843,#11182,.T.);
#27597=EDGE_CURVE('',#20841,#20919,#11183,.T.);
#27598=EDGE_CURVE('',#20920,#20839,#11184,.T.);
#27599=EDGE_CURVE('',#20837,#20920,#11185,.T.);
#27600=EDGE_CURVE('',#20921,#20835,#11186,.T.);
#27601=EDGE_CURVE('',#20833,#20921,#11187,.T.);
#27602=EDGE_CURVE('',#20922,#20831,#11188,.T.);
#27603=EDGE_CURVE('',#20829,#20922,#11189,.T.);
#27604=EDGE_CURVE('',#20923,#20827,#11190,.T.);
#27605=EDGE_CURVE('',#20819,#20923,#11191,.T.);
#27606=EDGE_CURVE('',#20924,#20822,#11192,.T.);
#27607=EDGE_CURVE('',#20825,#20924,#11193,.T.);
#27608=EDGE_CURVE('',#20925,#20823,#11194,.T.);
#27609=EDGE_CURVE('',#20817,#20925,#11195,.T.);
#27610=EDGE_CURVE('',#20926,#20815,#11196,.T.);
#27611=EDGE_CURVE('',#20813,#20926,#11197,.T.);
#27612=EDGE_CURVE('',#20927,#20811,#11198,.T.);
#27613=EDGE_CURVE('',#20809,#20927,#11199,.T.);
#27614=EDGE_CURVE('',#20928,#20807,#11200,.T.);
#27615=EDGE_CURVE('',#20805,#20928,#11201,.T.);
#27616=EDGE_CURVE('',#20929,#20803,#11202,.T.);
#27617=EDGE_CURVE('',#20801,#20929,#11203,.T.);
#27618=EDGE_CURVE('',#20930,#20799,#11204,.T.);
#27619=EDGE_CURVE('',#20797,#20930,#11205,.T.);
#27620=EDGE_CURVE('',#20931,#20795,#11206,.T.);
#27621=EDGE_CURVE('',#20793,#20931,#11207,.T.);
#27622=EDGE_CURVE('',#20932,#20791,#11208,.T.);
#27623=EDGE_CURVE('',#20789,#20932,#11209,.T.);
#27624=EDGE_CURVE('',#20933,#20787,#11210,.T.);
#27625=EDGE_CURVE('',#20785,#20933,#11211,.T.);
#27626=EDGE_CURVE('',#20934,#20783,#11212,.T.);
#27627=EDGE_CURVE('',#20781,#20934,#11213,.T.);
#27628=EDGE_CURVE('',#20935,#20779,#11214,.T.);
#27629=EDGE_CURVE('',#20763,#20935,#11215,.T.);
#27630=EDGE_CURVE('',#20936,#20766,#11216,.T.);
#27631=EDGE_CURVE('',#20767,#20936,#11217,.T.);
#27632=EDGE_CURVE('',#20937,#20770,#11218,.T.);
#27633=EDGE_CURVE('',#20771,#20937,#11219,.T.);
#27634=EDGE_CURVE('',#20938,#20774,#11220,.T.);
#27635=EDGE_CURVE('',#20777,#20938,#11221,.T.);
#27636=EDGE_CURVE('',#20939,#20775,#11222,.T.);
#27637=EDGE_CURVE('',#20761,#20939,#11223,.T.);
#27638=EDGE_CURVE('',#20940,#20759,#11224,.T.);
#27639=EDGE_CURVE('',#20757,#20940,#11225,.T.);
#27640=EDGE_CURVE('',#20941,#20755,#11226,.T.);
#27641=EDGE_CURVE('',#20753,#20941,#11227,.T.);
#27642=EDGE_CURVE('',#20942,#20751,#11228,.T.);
#27643=EDGE_CURVE('',#20749,#20942,#11229,.T.);
#27644=EDGE_CURVE('',#20943,#20747,#11230,.T.);
#27645=EDGE_CURVE('',#20745,#20943,#11231,.T.);
#27646=EDGE_CURVE('',#20944,#20743,#11232,.T.);
#27647=EDGE_CURVE('',#20741,#20944,#11233,.T.);
#27648=EDGE_CURVE('',#20945,#20739,#11234,.T.);
#27649=EDGE_CURVE('',#20737,#20945,#11235,.T.);
#27650=EDGE_CURVE('',#20946,#20735,#11236,.T.);
#27651=EDGE_CURVE('',#20733,#20946,#11237,.T.);
#27652=EDGE_CURVE('',#20947,#20731,#11238,.T.);
#27653=EDGE_CURVE('',#20729,#20947,#11239,.T.);
#27654=EDGE_CURVE('',#20948,#20727,#11240,.T.);
#27655=EDGE_CURVE('',#20725,#20948,#11241,.T.);
#27656=EDGE_CURVE('',#20949,#20723,#11242,.T.);
#27657=EDGE_CURVE('',#20721,#20949,#11243,.T.);
#27658=EDGE_CURVE('',#20950,#20719,#11244,.T.);
#27659=EDGE_CURVE('',#20717,#20950,#11245,.T.);
#27660=EDGE_CURVE('',#20951,#20715,#11246,.T.);
#27661=EDGE_CURVE('',#20713,#20951,#11247,.T.);
#27662=EDGE_CURVE('',#20952,#20711,#11248,.T.);
#27663=EDGE_CURVE('',#20709,#20952,#11249,.T.);
#27664=EDGE_CURVE('',#20953,#20707,#11250,.T.);
#27665=EDGE_CURVE('',#20705,#20953,#11251,.T.);
#27666=EDGE_CURVE('',#20954,#20700,#11252,.T.);
#27667=EDGE_CURVE('',#20704,#20954,#11253,.T.);
#27668=EDGE_CURVE('',#20955,#20706,#11254,.T.);
#27669=EDGE_CURVE('',#20708,#20955,#11255,.T.);
#27670=EDGE_CURVE('',#20956,#20710,#11256,.T.);
#27671=EDGE_CURVE('',#20712,#20956,#11257,.T.);
#27672=EDGE_CURVE('',#20957,#20714,#11258,.T.);
#27673=EDGE_CURVE('',#20716,#20957,#11259,.T.);
#27674=EDGE_CURVE('',#20958,#20718,#11260,.T.);
#27675=EDGE_CURVE('',#20720,#20958,#11261,.T.);
#27676=EDGE_CURVE('',#20959,#20722,#11262,.T.);
#27677=EDGE_CURVE('',#20724,#20959,#11263,.T.);
#27678=EDGE_CURVE('',#20960,#20726,#11264,.T.);
#27679=EDGE_CURVE('',#20728,#20960,#11265,.T.);
#27680=EDGE_CURVE('',#20961,#20730,#11266,.T.);
#27681=EDGE_CURVE('',#20732,#20961,#11267,.T.);
#27682=EDGE_CURVE('',#20962,#20734,#11268,.T.);
#27683=EDGE_CURVE('',#20736,#20962,#11269,.T.);
#27684=EDGE_CURVE('',#20963,#20738,#11270,.T.);
#27685=EDGE_CURVE('',#20740,#20963,#11271,.T.);
#27686=EDGE_CURVE('',#20964,#20742,#11272,.T.);
#27687=EDGE_CURVE('',#20744,#20964,#11273,.T.);
#27688=EDGE_CURVE('',#20965,#20746,#11274,.T.);
#27689=EDGE_CURVE('',#20748,#20965,#11275,.T.);
#27690=EDGE_CURVE('',#20966,#20750,#11276,.T.);
#27691=EDGE_CURVE('',#20752,#20966,#11277,.T.);
#27692=EDGE_CURVE('',#20967,#20754,#11278,.T.);
#27693=EDGE_CURVE('',#20756,#20967,#11279,.T.);
#27694=EDGE_CURVE('',#20968,#20758,#11280,.T.);
#27695=EDGE_CURVE('',#20760,#20968,#11281,.T.);
#27696=EDGE_CURVE('',#20969,#20762,#11282,.T.);
#27697=EDGE_CURVE('',#20776,#20969,#11283,.T.);
#27698=EDGE_CURVE('',#20970,#20778,#11284,.T.);
#27699=EDGE_CURVE('',#20773,#20970,#11285,.T.);
#27700=EDGE_CURVE('',#20971,#20772,#11286,.T.);
#27701=EDGE_CURVE('',#20769,#20971,#11287,.T.);
#27702=EDGE_CURVE('',#20972,#20768,#11288,.T.);
#27703=EDGE_CURVE('',#20765,#20972,#11289,.T.);
#27704=EDGE_CURVE('',#20973,#20764,#11290,.T.);
#27705=EDGE_CURVE('',#20780,#20973,#11291,.T.);
#27706=EDGE_CURVE('',#20974,#20782,#11292,.T.);
#27707=EDGE_CURVE('',#20784,#20974,#11293,.T.);
#27708=EDGE_CURVE('',#20975,#20786,#11294,.T.);
#27709=EDGE_CURVE('',#20788,#20975,#11295,.T.);
#27710=EDGE_CURVE('',#20976,#20790,#11296,.T.);
#27711=EDGE_CURVE('',#20792,#20976,#11297,.T.);
#27712=EDGE_CURVE('',#20977,#20794,#11298,.T.);
#27713=EDGE_CURVE('',#20796,#20977,#11299,.T.);
#27714=EDGE_CURVE('',#20978,#20798,#11300,.T.);
#27715=EDGE_CURVE('',#20800,#20978,#11301,.T.);
#27716=EDGE_CURVE('',#20979,#20802,#11302,.T.);
#27717=EDGE_CURVE('',#20804,#20979,#11303,.T.);
#27718=EDGE_CURVE('',#20980,#20806,#11304,.T.);
#27719=EDGE_CURVE('',#20808,#20980,#11305,.T.);
#27720=EDGE_CURVE('',#20981,#20810,#11306,.T.);
#27721=EDGE_CURVE('',#20812,#20981,#11307,.T.);
#27722=EDGE_CURVE('',#20982,#20814,#11308,.T.);
#27723=EDGE_CURVE('',#20816,#20982,#11309,.T.);
#27724=EDGE_CURVE('',#20983,#20818,#11310,.T.);
#27725=EDGE_CURVE('',#20824,#20983,#11311,.T.);
#27726=EDGE_CURVE('',#20984,#20826,#11312,.T.);
#27727=EDGE_CURVE('',#20821,#20984,#11313,.T.);
#27728=EDGE_CURVE('',#20985,#20820,#11314,.T.);
#27729=EDGE_CURVE('',#20828,#20985,#11315,.T.);
#27730=EDGE_CURVE('',#20986,#20830,#11316,.T.);
#27731=EDGE_CURVE('',#20832,#20986,#11317,.T.);
#27732=EDGE_CURVE('',#20987,#20834,#11318,.T.);
#27733=EDGE_CURVE('',#20836,#20987,#11319,.T.);
#27734=EDGE_CURVE('',#20988,#20838,#11320,.T.);
#27735=EDGE_CURVE('',#20840,#20988,#11321,.T.);
#27736=EDGE_CURVE('',#20989,#20842,#11322,.T.);
#27737=EDGE_CURVE('',#20844,#20989,#11323,.T.);
#27738=EDGE_CURVE('',#20990,#20846,#11324,.T.);
#27739=EDGE_CURVE('',#20848,#20990,#11325,.T.);
#27740=EDGE_CURVE('',#20991,#20850,#11326,.T.);
#27741=EDGE_CURVE('',#20852,#20991,#11327,.T.);
#27742=EDGE_CURVE('',#20992,#20854,#11328,.T.);
#27743=EDGE_CURVE('',#20856,#20992,#11329,.T.);
#27744=EDGE_CURVE('',#20993,#20858,#11330,.T.);
#27745=EDGE_CURVE('',#20888,#20993,#11331,.T.);
#27746=EDGE_CURVE('',#20994,#20890,#11332,.T.);
#27747=EDGE_CURVE('',#20885,#20994,#11333,.T.);
#27748=EDGE_CURVE('',#20995,#20884,#11334,.T.);
#27749=EDGE_CURVE('',#20881,#20995,#11335,.T.);
#27750=EDGE_CURVE('',#20996,#20880,#11336,.T.);
#27751=EDGE_CURVE('',#20877,#20996,#11337,.T.);
#27752=EDGE_CURVE('',#20997,#20876,#11338,.T.);
#27753=EDGE_CURVE('',#20873,#20997,#11339,.T.);
#27754=EDGE_CURVE('',#20998,#20872,#11340,.T.);
#27755=EDGE_CURVE('',#20869,#20998,#11341,.T.);
#27756=EDGE_CURVE('',#20999,#20868,#11342,.T.);
#27757=EDGE_CURVE('',#20865,#20999,#11343,.T.);
#27758=EDGE_CURVE('',#21000,#20864,#11344,.T.);
#27759=EDGE_CURVE('',#20861,#21000,#11345,.T.);
#27760=EDGE_CURVE('',#21001,#20860,#11346,.T.);
#27761=EDGE_CURVE('',#20892,#21001,#11347,.T.);
#27762=EDGE_CURVE('',#21002,#20894,#11348,.T.);
#27763=EDGE_CURVE('',#20900,#21002,#11349,.T.);
#27764=EDGE_CURVE('',#21003,#20902,#11350,.T.);
#27765=EDGE_CURVE('',#20897,#21003,#11351,.T.);
#27766=EDGE_CURVE('',#21004,#20896,#11352,.T.);
#27767=EDGE_CURVE('',#20701,#21004,#11353,.T.);
#27768=EDGE_CURVE('',#20905,#21003,#11354,.T.);
#27769=EDGE_CURVE('',#20904,#21004,#11355,.T.);
#27770=EDGE_CURVE('',#20906,#21002,#11356,.T.);
#27771=EDGE_CURVE('',#20914,#20994,#11357,.T.);
#27772=EDGE_CURVE('',#20913,#20995,#11358,.T.);
#27773=EDGE_CURVE('',#20912,#20996,#11359,.T.);
#27774=EDGE_CURVE('',#20911,#20997,#11360,.T.);
#27775=EDGE_CURVE('',#20910,#20998,#11361,.T.);
#27776=EDGE_CURVE('',#20909,#20999,#11362,.T.);
#27777=EDGE_CURVE('',#20908,#21000,#11363,.T.);
#27778=EDGE_CURVE('',#20907,#21001,#11364,.T.);
#27779=EDGE_CURVE('',#20915,#20993,#11365,.T.);
#27780=EDGE_CURVE('',#20916,#20992,#11366,.T.);
#27781=EDGE_CURVE('',#20917,#20991,#11367,.T.);
#27782=EDGE_CURVE('',#20918,#20990,#11368,.T.);
#27783=EDGE_CURVE('',#20919,#20989,#11369,.T.);
#27784=EDGE_CURVE('',#20920,#20988,#11370,.T.);
#27785=EDGE_CURVE('',#20921,#20987,#11371,.T.);
#27786=EDGE_CURVE('',#20922,#20986,#11372,.T.);
#27787=EDGE_CURVE('',#20924,#20984,#11373,.T.);
#27788=EDGE_CURVE('',#20923,#20985,#11374,.T.);
#27789=EDGE_CURVE('',#20925,#20983,#11375,.T.);
#27790=EDGE_CURVE('',#20926,#20982,#11376,.T.);
#27791=EDGE_CURVE('',#20927,#20981,#11377,.T.);
#27792=EDGE_CURVE('',#20928,#20980,#11378,.T.);
#27793=EDGE_CURVE('',#20929,#20979,#11379,.T.);
#27794=EDGE_CURVE('',#20930,#20978,#11380,.T.);
#27795=EDGE_CURVE('',#20931,#20977,#11381,.T.);
#27796=EDGE_CURVE('',#20932,#20976,#11382,.T.);
#27797=EDGE_CURVE('',#20933,#20975,#11383,.T.);
#27798=EDGE_CURVE('',#20934,#20974,#11384,.T.);
#27799=EDGE_CURVE('',#20938,#20970,#11385,.T.);
#27800=EDGE_CURVE('',#20937,#20971,#11386,.T.);
#27801=EDGE_CURVE('',#20936,#20972,#11387,.T.);
#27802=EDGE_CURVE('',#20935,#20973,#11388,.T.);
#27803=EDGE_CURVE('',#20939,#20969,#11389,.T.);
#27804=EDGE_CURVE('',#20940,#20968,#11390,.T.);
#27805=EDGE_CURVE('',#20941,#20967,#11391,.T.);
#27806=EDGE_CURVE('',#20942,#20966,#11392,.T.);
#27807=EDGE_CURVE('',#20943,#20965,#11393,.T.);
#27808=EDGE_CURVE('',#20944,#20964,#11394,.T.);
#27809=EDGE_CURVE('',#20945,#20963,#11395,.T.);
#27810=EDGE_CURVE('',#20946,#20962,#11396,.T.);
#27811=EDGE_CURVE('',#20947,#20961,#11397,.T.);
#27812=EDGE_CURVE('',#20948,#20960,#11398,.T.);
#27813=EDGE_CURVE('',#20949,#20959,#11399,.T.);
#27814=EDGE_CURVE('',#20950,#20958,#11400,.T.);
#27815=EDGE_CURVE('',#20951,#20957,#11401,.T.);
#27816=EDGE_CURVE('',#20952,#20956,#11402,.T.);
#27817=EDGE_CURVE('',#20953,#20955,#11403,.T.);
#27818=EDGE_CURVE('',#20903,#20954,#11404,.T.);
#40412=ORIENTED_EDGE('',*,*,#27348,.T.);
#40413=ORIENTED_EDGE('',*,*,#27349,.T.);
#40414=ORIENTED_EDGE('',*,*,#27350,.F.);
#40415=ORIENTED_EDGE('',*,*,#27349,.F.);
#40416=ORIENTED_EDGE('',*,*,#27351,.T.);
#40417=ORIENTED_EDGE('',*,*,#27352,.T.);
#40418=ORIENTED_EDGE('',*,*,#27353,.F.);
#40419=ORIENTED_EDGE('',*,*,#27352,.F.);
#40420=ORIENTED_EDGE('',*,*,#27354,.F.);
#40421=ORIENTED_EDGE('',*,*,#27355,.T.);
#40422=ORIENTED_EDGE('',*,*,#27356,.T.);
#40423=ORIENTED_EDGE('',*,*,#27355,.F.);
#40424=ORIENTED_EDGE('',*,*,#27357,.F.);
#40425=ORIENTED_EDGE('',*,*,#27358,.T.);
#40426=ORIENTED_EDGE('',*,*,#27359,.T.);
#40427=ORIENTED_EDGE('',*,*,#27358,.F.);
#40428=ORIENTED_EDGE('',*,*,#27360,.T.);
#40429=ORIENTED_EDGE('',*,*,#27361,.F.);
#40430=ORIENTED_EDGE('',*,*,#27362,.F.);
#40431=ORIENTED_EDGE('',*,*,#27363,.T.);
#40432=ORIENTED_EDGE('',*,*,#27364,.F.);
#40433=ORIENTED_EDGE('',*,*,#27365,.T.);
#40434=ORIENTED_EDGE('',*,*,#27366,.T.);
#40435=ORIENTED_EDGE('',*,*,#27367,.F.);
#40436=ORIENTED_EDGE('',*,*,#27368,.F.);
#40437=ORIENTED_EDGE('',*,*,#27369,.T.);
#40438=ORIENTED_EDGE('',*,*,#27370,.T.);
#40439=ORIENTED_EDGE('',*,*,#27371,.F.);
#40440=ORIENTED_EDGE('',*,*,#27372,.F.);
#40441=ORIENTED_EDGE('',*,*,#27373,.T.);
#40442=ORIENTED_EDGE('',*,*,#27374,.T.);
#40443=ORIENTED_EDGE('',*,*,#27375,.F.);
#40444=ORIENTED_EDGE('',*,*,#27376,.F.);
#40445=ORIENTED_EDGE('',*,*,#27377,.T.);
#40446=ORIENTED_EDGE('',*,*,#27378,.T.);
#40447=ORIENTED_EDGE('',*,*,#27379,.F.);
#40448=ORIENTED_EDGE('',*,*,#27380,.F.);
#40449=ORIENTED_EDGE('',*,*,#27381,.T.);
#40450=ORIENTED_EDGE('',*,*,#27382,.T.);
#40451=ORIENTED_EDGE('',*,*,#27383,.F.);
#40452=ORIENTED_EDGE('',*,*,#27384,.F.);
#40453=ORIENTED_EDGE('',*,*,#27385,.T.);
#40454=ORIENTED_EDGE('',*,*,#27386,.T.);
#40455=ORIENTED_EDGE('',*,*,#27387,.F.);
#40456=ORIENTED_EDGE('',*,*,#27388,.F.);
#40457=ORIENTED_EDGE('',*,*,#27389,.T.);
#40458=ORIENTED_EDGE('',*,*,#27390,.T.);
#40459=ORIENTED_EDGE('',*,*,#27391,.F.);
#40460=ORIENTED_EDGE('',*,*,#27392,.F.);
#40461=ORIENTED_EDGE('',*,*,#27393,.T.);
#40462=ORIENTED_EDGE('',*,*,#27394,.T.);
#40463=ORIENTED_EDGE('',*,*,#27395,.F.);
#40464=ORIENTED_EDGE('',*,*,#27396,.F.);
#40465=ORIENTED_EDGE('',*,*,#27397,.T.);
#40466=ORIENTED_EDGE('',*,*,#27398,.T.);
#40467=ORIENTED_EDGE('',*,*,#27399,.F.);
#40468=ORIENTED_EDGE('',*,*,#27400,.F.);
#40469=ORIENTED_EDGE('',*,*,#27401,.T.);
#40470=ORIENTED_EDGE('',*,*,#27402,.T.);
#40471=ORIENTED_EDGE('',*,*,#27403,.F.);
#40472=ORIENTED_EDGE('',*,*,#27404,.F.);
#40473=ORIENTED_EDGE('',*,*,#27405,.T.);
#40474=ORIENTED_EDGE('',*,*,#27406,.T.);
#40475=ORIENTED_EDGE('',*,*,#27407,.F.);
#40476=ORIENTED_EDGE('',*,*,#27408,.F.);
#40477=ORIENTED_EDGE('',*,*,#27409,.T.);
#40478=ORIENTED_EDGE('',*,*,#27410,.T.);
#40479=ORIENTED_EDGE('',*,*,#27411,.F.);
#40480=ORIENTED_EDGE('',*,*,#27412,.F.);
#40481=ORIENTED_EDGE('',*,*,#27413,.T.);
#40482=ORIENTED_EDGE('',*,*,#27414,.T.);
#40483=ORIENTED_EDGE('',*,*,#27415,.F.);
#40484=ORIENTED_EDGE('',*,*,#27416,.F.);
#40485=ORIENTED_EDGE('',*,*,#27417,.T.);
#40486=ORIENTED_EDGE('',*,*,#27418,.T.);
#40487=ORIENTED_EDGE('',*,*,#27419,.F.);
#40488=ORIENTED_EDGE('',*,*,#27420,.F.);
#40489=ORIENTED_EDGE('',*,*,#27421,.T.);
#40490=ORIENTED_EDGE('',*,*,#27422,.T.);
#40491=ORIENTED_EDGE('',*,*,#27423,.F.);
#40492=ORIENTED_EDGE('',*,*,#27424,.T.);
#40493=ORIENTED_EDGE('',*,*,#27425,.F.);
#40494=ORIENTED_EDGE('',*,*,#27426,.F.);
#40495=ORIENTED_EDGE('',*,*,#27427,.T.);
#40496=ORIENTED_EDGE('',*,*,#27428,.T.);
#40497=ORIENTED_EDGE('',*,*,#27429,.F.);
#40498=ORIENTED_EDGE('',*,*,#27430,.F.);
#40499=ORIENTED_EDGE('',*,*,#27431,.T.);
#40500=ORIENTED_EDGE('',*,*,#27432,.T.);
#40501=ORIENTED_EDGE('',*,*,#27433,.F.);
#40502=ORIENTED_EDGE('',*,*,#27434,.F.);
#40503=ORIENTED_EDGE('',*,*,#27435,.T.);
#40504=ORIENTED_EDGE('',*,*,#27436,.F.);
#40505=ORIENTED_EDGE('',*,*,#27437,.T.);
#40506=ORIENTED_EDGE('',*,*,#27438,.T.);
#40507=ORIENTED_EDGE('',*,*,#27439,.F.);
#40508=ORIENTED_EDGE('',*,*,#27440,.F.);
#40509=ORIENTED_EDGE('',*,*,#27441,.T.);
#40510=ORIENTED_EDGE('',*,*,#27442,.T.);
#40511=ORIENTED_EDGE('',*,*,#27443,.F.);
#40512=ORIENTED_EDGE('',*,*,#27444,.F.);
#40513=ORIENTED_EDGE('',*,*,#27445,.T.);
#40514=ORIENTED_EDGE('',*,*,#27446,.T.);
#40515=ORIENTED_EDGE('',*,*,#27447,.F.);
#40516=ORIENTED_EDGE('',*,*,#27448,.F.);
#40517=ORIENTED_EDGE('',*,*,#27449,.T.);
#40518=ORIENTED_EDGE('',*,*,#27450,.T.);
#40519=ORIENTED_EDGE('',*,*,#27451,.F.);
#40520=ORIENTED_EDGE('',*,*,#27452,.F.);
#40521=ORIENTED_EDGE('',*,*,#27453,.T.);
#40522=ORIENTED_EDGE('',*,*,#27454,.T.);
#40523=ORIENTED_EDGE('',*,*,#27455,.F.);
#40524=ORIENTED_EDGE('',*,*,#27456,.F.);
#40525=ORIENTED_EDGE('',*,*,#27457,.T.);
#40526=ORIENTED_EDGE('',*,*,#27458,.T.);
#40527=ORIENTED_EDGE('',*,*,#27459,.F.);
#40528=ORIENTED_EDGE('',*,*,#27460,.F.);
#40529=ORIENTED_EDGE('',*,*,#27461,.T.);
#40530=ORIENTED_EDGE('',*,*,#27462,.T.);
#40531=ORIENTED_EDGE('',*,*,#27463,.F.);
#40532=ORIENTED_EDGE('',*,*,#27464,.F.);
#40533=ORIENTED_EDGE('',*,*,#27465,.T.);
#40534=ORIENTED_EDGE('',*,*,#27466,.T.);
#40535=ORIENTED_EDGE('',*,*,#27467,.F.);
#40536=ORIENTED_EDGE('',*,*,#27468,.F.);
#40537=ORIENTED_EDGE('',*,*,#27469,.T.);
#40538=ORIENTED_EDGE('',*,*,#27470,.T.);
#40539=ORIENTED_EDGE('',*,*,#27471,.F.);
#40540=ORIENTED_EDGE('',*,*,#27472,.F.);
#40541=ORIENTED_EDGE('',*,*,#27473,.T.);
#40542=ORIENTED_EDGE('',*,*,#27474,.T.);
#40543=ORIENTED_EDGE('',*,*,#27475,.F.);
#40544=ORIENTED_EDGE('',*,*,#27476,.F.);
#40545=ORIENTED_EDGE('',*,*,#27477,.T.);
#40546=ORIENTED_EDGE('',*,*,#27478,.T.);
#40547=ORIENTED_EDGE('',*,*,#27479,.F.);
#40548=ORIENTED_EDGE('',*,*,#27480,.T.);
#40549=ORIENTED_EDGE('',*,*,#27481,.F.);
#40550=ORIENTED_EDGE('',*,*,#27482,.F.);
#40551=ORIENTED_EDGE('',*,*,#27483,.T.);
#40552=ORIENTED_EDGE('',*,*,#27484,.F.);
#40553=ORIENTED_EDGE('',*,*,#27485,.T.);
#40554=ORIENTED_EDGE('',*,*,#27486,.T.);
#40555=ORIENTED_EDGE('',*,*,#27487,.F.);
#40556=ORIENTED_EDGE('',*,*,#27488,.F.);
#40557=ORIENTED_EDGE('',*,*,#27489,.T.);
#40558=ORIENTED_EDGE('',*,*,#27490,.T.);
#40559=ORIENTED_EDGE('',*,*,#27491,.F.);
#40560=ORIENTED_EDGE('',*,*,#27492,.F.);
#40561=ORIENTED_EDGE('',*,*,#27493,.T.);
#40562=ORIENTED_EDGE('',*,*,#27494,.T.);
#40563=ORIENTED_EDGE('',*,*,#27495,.F.);
#40564=ORIENTED_EDGE('',*,*,#27496,.F.);
#40565=ORIENTED_EDGE('',*,*,#27497,.T.);
#40566=ORIENTED_EDGE('',*,*,#27498,.T.);
#40567=ORIENTED_EDGE('',*,*,#27499,.F.);
#40568=ORIENTED_EDGE('',*,*,#27500,.F.);
#40569=ORIENTED_EDGE('',*,*,#27501,.T.);
#40570=ORIENTED_EDGE('',*,*,#27502,.T.);
#40571=ORIENTED_EDGE('',*,*,#27503,.F.);
#40572=ORIENTED_EDGE('',*,*,#27504,.F.);
#40573=ORIENTED_EDGE('',*,*,#27505,.T.);
#40574=ORIENTED_EDGE('',*,*,#27506,.T.);
#40575=ORIENTED_EDGE('',*,*,#27507,.F.);
#40576=ORIENTED_EDGE('',*,*,#27508,.F.);
#40577=ORIENTED_EDGE('',*,*,#27509,.T.);
#40578=ORIENTED_EDGE('',*,*,#27510,.T.);
#40579=ORIENTED_EDGE('',*,*,#27511,.F.);
#40580=ORIENTED_EDGE('',*,*,#27512,.F.);
#40581=ORIENTED_EDGE('',*,*,#27513,.T.);
#40582=ORIENTED_EDGE('',*,*,#27514,.T.);
#40583=ORIENTED_EDGE('',*,*,#27515,.F.);
#40584=ORIENTED_EDGE('',*,*,#27516,.F.);
#40585=ORIENTED_EDGE('',*,*,#27517,.T.);
#40586=ORIENTED_EDGE('',*,*,#27518,.T.);
#40587=ORIENTED_EDGE('',*,*,#27519,.F.);
#40588=ORIENTED_EDGE('',*,*,#27520,.T.);
#40589=ORIENTED_EDGE('',*,*,#27521,.F.);
#40590=ORIENTED_EDGE('',*,*,#27522,.F.);
#40591=ORIENTED_EDGE('',*,*,#27523,.T.);
#40592=ORIENTED_EDGE('',*,*,#27524,.T.);
#40593=ORIENTED_EDGE('',*,*,#27525,.F.);
#40594=ORIENTED_EDGE('',*,*,#27526,.F.);
#40595=ORIENTED_EDGE('',*,*,#27527,.T.);
#40596=ORIENTED_EDGE('',*,*,#27528,.T.);
#40597=ORIENTED_EDGE('',*,*,#27529,.F.);
#40598=ORIENTED_EDGE('',*,*,#27530,.F.);
#40599=ORIENTED_EDGE('',*,*,#27531,.T.);
#40600=ORIENTED_EDGE('',*,*,#27532,.T.);
#40601=ORIENTED_EDGE('',*,*,#27533,.F.);
#40602=ORIENTED_EDGE('',*,*,#27534,.F.);
#40603=ORIENTED_EDGE('',*,*,#27535,.T.);
#40604=ORIENTED_EDGE('',*,*,#27536,.T.);
#40605=ORIENTED_EDGE('',*,*,#27537,.F.);
#40606=ORIENTED_EDGE('',*,*,#27538,.F.);
#40607=ORIENTED_EDGE('',*,*,#27539,.T.);
#40608=ORIENTED_EDGE('',*,*,#27540,.T.);
#40609=ORIENTED_EDGE('',*,*,#27541,.F.);
#40610=ORIENTED_EDGE('',*,*,#27542,.F.);
#40611=ORIENTED_EDGE('',*,*,#27543,.T.);
#40612=ORIENTED_EDGE('',*,*,#27544,.T.);
#40613=ORIENTED_EDGE('',*,*,#27545,.F.);
#40614=ORIENTED_EDGE('',*,*,#27546,.F.);
#40615=ORIENTED_EDGE('',*,*,#27547,.T.);
#40616=ORIENTED_EDGE('',*,*,#27548,.F.);
#40617=ORIENTED_EDGE('',*,*,#27549,.T.);
#40618=ORIENTED_EDGE('',*,*,#27550,.T.);
#40619=ORIENTED_EDGE('',*,*,#27551,.F.);
#40620=ORIENTED_EDGE('',*,*,#27552,.F.);
#40621=ORIENTED_EDGE('',*,*,#27553,.T.);
#40622=ORIENTED_EDGE('',*,*,#27554,.T.);
#40623=ORIENTED_EDGE('',*,*,#27555,.F.);
#40624=ORIENTED_EDGE('',*,*,#27556,.T.);
#40625=ORIENTED_EDGE('',*,*,#27557,.F.);
#40626=ORIENTED_EDGE('',*,*,#27558,.F.);
#40627=ORIENTED_EDGE('',*,*,#27559,.T.);
#40628=ORIENTED_EDGE('',*,*,#27560,.F.);
#40629=ORIENTED_EDGE('',*,*,#27561,.T.);
#40630=ORIENTED_EDGE('',*,*,#27562,.T.);
#40631=ORIENTED_EDGE('',*,*,#27563,.F.);
#40632=ORIENTED_EDGE('',*,*,#27564,.F.);
#40633=ORIENTED_EDGE('',*,*,#27565,.F.);
#40634=ORIENTED_EDGE('',*,*,#27363,.F.);
#40635=ORIENTED_EDGE('',*,*,#27566,.F.);
#40636=ORIENTED_EDGE('',*,*,#27567,.F.);
#40637=ORIENTED_EDGE('',*,*,#27559,.F.);
#40638=ORIENTED_EDGE('',*,*,#27568,.F.);
#40639=ORIENTED_EDGE('',*,*,#27569,.F.);
#40640=ORIENTED_EDGE('',*,*,#27561,.F.);
#40641=ORIENTED_EDGE('',*,*,#27570,.F.);
#40642=ORIENTED_EDGE('',*,*,#27571,.F.);
#40643=ORIENTED_EDGE('',*,*,#27553,.F.);
#40644=ORIENTED_EDGE('',*,*,#27572,.F.);
#40645=ORIENTED_EDGE('',*,*,#27573,.F.);
#40646=ORIENTED_EDGE('',*,*,#27523,.F.);
#40647=ORIENTED_EDGE('',*,*,#27574,.F.);
#40648=ORIENTED_EDGE('',*,*,#27575,.F.);
#40649=ORIENTED_EDGE('',*,*,#27527,.F.);
#40650=ORIENTED_EDGE('',*,*,#27576,.F.);
#40651=ORIENTED_EDGE('',*,*,#27577,.F.);
#40652=ORIENTED_EDGE('',*,*,#27531,.F.);
#40653=ORIENTED_EDGE('',*,*,#27578,.F.);
#40654=ORIENTED_EDGE('',*,*,#27579,.F.);
#40655=ORIENTED_EDGE('',*,*,#27535,.F.);
#40656=ORIENTED_EDGE('',*,*,#27580,.F.);
#40657=ORIENTED_EDGE('',*,*,#27581,.F.);
#40658=ORIENTED_EDGE('',*,*,#27539,.F.);
#40659=ORIENTED_EDGE('',*,*,#27582,.F.);
#40660=ORIENTED_EDGE('',*,*,#27583,.F.);
#40661=ORIENTED_EDGE('',*,*,#27543,.F.);
#40662=ORIENTED_EDGE('',*,*,#27584,.F.);
#40663=ORIENTED_EDGE('',*,*,#27585,.F.);
#40664=ORIENTED_EDGE('',*,*,#27547,.F.);
#40665=ORIENTED_EDGE('',*,*,#27586,.F.);
#40666=ORIENTED_EDGE('',*,*,#27587,.F.);
#40667=ORIENTED_EDGE('',*,*,#27549,.F.);
#40668=ORIENTED_EDGE('',*,*,#27588,.F.);
#40669=ORIENTED_EDGE('',*,*,#27589,.F.);
#40670=ORIENTED_EDGE('',*,*,#27517,.F.);
#40671=ORIENTED_EDGE('',*,*,#27590,.F.);
#40672=ORIENTED_EDGE('',*,*,#27591,.F.);
#40673=ORIENTED_EDGE('',*,*,#27513,.F.);
#40674=ORIENTED_EDGE('',*,*,#27592,.F.);
#40675=ORIENTED_EDGE('',*,*,#27593,.F.);
#40676=ORIENTED_EDGE('',*,*,#27509,.F.);
#40677=ORIENTED_EDGE('',*,*,#27594,.F.);
#40678=ORIENTED_EDGE('',*,*,#27595,.F.);
#40679=ORIENTED_EDGE('',*,*,#27505,.F.);
#40680=ORIENTED_EDGE('',*,*,#27596,.F.);
#40681=ORIENTED_EDGE('',*,*,#27597,.F.);
#40682=ORIENTED_EDGE('',*,*,#27501,.F.);
#40683=ORIENTED_EDGE('',*,*,#27598,.F.);
#40684=ORIENTED_EDGE('',*,*,#27599,.F.);
#40685=ORIENTED_EDGE('',*,*,#27497,.F.);
#40686=ORIENTED_EDGE('',*,*,#27600,.F.);
#40687=ORIENTED_EDGE('',*,*,#27601,.F.);
#40688=ORIENTED_EDGE('',*,*,#27493,.F.);
#40689=ORIENTED_EDGE('',*,*,#27602,.F.);
#40690=ORIENTED_EDGE('',*,*,#27603,.F.);
#40691=ORIENTED_EDGE('',*,*,#27489,.F.);
#40692=ORIENTED_EDGE('',*,*,#27604,.F.);
#40693=ORIENTED_EDGE('',*,*,#27605,.F.);
#40694=ORIENTED_EDGE('',*,*,#27483,.F.);
#40695=ORIENTED_EDGE('',*,*,#27606,.F.);
#40696=ORIENTED_EDGE('',*,*,#27607,.F.);
#40697=ORIENTED_EDGE('',*,*,#27485,.F.);
#40698=ORIENTED_EDGE('',*,*,#27608,.F.);
#40699=ORIENTED_EDGE('',*,*,#27609,.F.);
#40700=ORIENTED_EDGE('',*,*,#27477,.F.);
#40701=ORIENTED_EDGE('',*,*,#27610,.F.);
#40702=ORIENTED_EDGE('',*,*,#27611,.F.);
#40703=ORIENTED_EDGE('',*,*,#27473,.F.);
#40704=ORIENTED_EDGE('',*,*,#27612,.F.);
#40705=ORIENTED_EDGE('',*,*,#27613,.F.);
#40706=ORIENTED_EDGE('',*,*,#27469,.F.);
#40707=ORIENTED_EDGE('',*,*,#27614,.F.);
#40708=ORIENTED_EDGE('',*,*,#27615,.F.);
#40709=ORIENTED_EDGE('',*,*,#27465,.F.);
#40710=ORIENTED_EDGE('',*,*,#27616,.F.);
#40711=ORIENTED_EDGE('',*,*,#27617,.F.);
#40712=ORIENTED_EDGE('',*,*,#27461,.F.);
#40713=ORIENTED_EDGE('',*,*,#27618,.F.);
#40714=ORIENTED_EDGE('',*,*,#27619,.F.);
#40715=ORIENTED_EDGE('',*,*,#27457,.F.);
#40716=ORIENTED_EDGE('',*,*,#27620,.F.);
#40717=ORIENTED_EDGE('',*,*,#27621,.F.);
#40718=ORIENTED_EDGE('',*,*,#27453,.F.);
#40719=ORIENTED_EDGE('',*,*,#27622,.F.);
#40720=ORIENTED_EDGE('',*,*,#27623,.F.);
#40721=ORIENTED_EDGE('',*,*,#27449,.F.);
#40722=ORIENTED_EDGE('',*,*,#27624,.F.);
#40723=ORIENTED_EDGE('',*,*,#27625,.F.);
#40724=ORIENTED_EDGE('',*,*,#27445,.F.);
#40725=ORIENTED_EDGE('',*,*,#27626,.F.);
#40726=ORIENTED_EDGE('',*,*,#27627,.F.);
#40727=ORIENTED_EDGE('',*,*,#27441,.F.);
#40728=ORIENTED_EDGE('',*,*,#27628,.F.);
#40729=ORIENTED_EDGE('',*,*,#27629,.F.);
#40730=ORIENTED_EDGE('',*,*,#27427,.F.);
#40731=ORIENTED_EDGE('',*,*,#27630,.F.);
#40732=ORIENTED_EDGE('',*,*,#27631,.F.);
#40733=ORIENTED_EDGE('',*,*,#27431,.F.);
#40734=ORIENTED_EDGE('',*,*,#27632,.F.);
#40735=ORIENTED_EDGE('',*,*,#27633,.F.);
#40736=ORIENTED_EDGE('',*,*,#27435,.F.);
#40737=ORIENTED_EDGE('',*,*,#27634,.F.);
#40738=ORIENTED_EDGE('',*,*,#27635,.F.);
#40739=ORIENTED_EDGE('',*,*,#27437,.F.);
#40740=ORIENTED_EDGE('',*,*,#27636,.F.);
#40741=ORIENTED_EDGE('',*,*,#27637,.F.);
#40742=ORIENTED_EDGE('',*,*,#27421,.F.);
#40743=ORIENTED_EDGE('',*,*,#27638,.F.);
#40744=ORIENTED_EDGE('',*,*,#27639,.F.);
#40745=ORIENTED_EDGE('',*,*,#27417,.F.);
#40746=ORIENTED_EDGE('',*,*,#27640,.F.);
#40747=ORIENTED_EDGE('',*,*,#27641,.F.);
#40748=ORIENTED_EDGE('',*,*,#27413,.F.);
#40749=ORIENTED_EDGE('',*,*,#27642,.F.);
#40750=ORIENTED_EDGE('',*,*,#27643,.F.);
#40751=ORIENTED_EDGE('',*,*,#27409,.F.);
#40752=ORIENTED_EDGE('',*,*,#27644,.F.);
#40753=ORIENTED_EDGE('',*,*,#27645,.F.);
#40754=ORIENTED_EDGE('',*,*,#27405,.F.);
#40755=ORIENTED_EDGE('',*,*,#27646,.F.);
#40756=ORIENTED_EDGE('',*,*,#27647,.F.);
#40757=ORIENTED_EDGE('',*,*,#27401,.F.);
#40758=ORIENTED_EDGE('',*,*,#27648,.F.);
#40759=ORIENTED_EDGE('',*,*,#27649,.F.);
#40760=ORIENTED_EDGE('',*,*,#27397,.F.);
#40761=ORIENTED_EDGE('',*,*,#27650,.F.);
#40762=ORIENTED_EDGE('',*,*,#27651,.F.);
#40763=ORIENTED_EDGE('',*,*,#27393,.F.);
#40764=ORIENTED_EDGE('',*,*,#27652,.F.);
#40765=ORIENTED_EDGE('',*,*,#27653,.F.);
#40766=ORIENTED_EDGE('',*,*,#27389,.F.);
#40767=ORIENTED_EDGE('',*,*,#27654,.F.);
#40768=ORIENTED_EDGE('',*,*,#27655,.F.);
#40769=ORIENTED_EDGE('',*,*,#27385,.F.);
#40770=ORIENTED_EDGE('',*,*,#27656,.F.);
#40771=ORIENTED_EDGE('',*,*,#27657,.F.);
#40772=ORIENTED_EDGE('',*,*,#27381,.F.);
#40773=ORIENTED_EDGE('',*,*,#27658,.F.);
#40774=ORIENTED_EDGE('',*,*,#27659,.F.);
#40775=ORIENTED_EDGE('',*,*,#27377,.F.);
#40776=ORIENTED_EDGE('',*,*,#27660,.F.);
#40777=ORIENTED_EDGE('',*,*,#27661,.F.);
#40778=ORIENTED_EDGE('',*,*,#27373,.F.);
#40779=ORIENTED_EDGE('',*,*,#27662,.F.);
#40780=ORIENTED_EDGE('',*,*,#27663,.F.);
#40781=ORIENTED_EDGE('',*,*,#27369,.F.);
#40782=ORIENTED_EDGE('',*,*,#27664,.F.);
#40783=ORIENTED_EDGE('',*,*,#27665,.F.);
#40784=ORIENTED_EDGE('',*,*,#27365,.F.);
#40785=ORIENTED_EDGE('',*,*,#27356,.F.);
#40786=ORIENTED_EDGE('',*,*,#27666,.F.);
#40787=ORIENTED_EDGE('',*,*,#27667,.F.);
#40788=ORIENTED_EDGE('',*,*,#27367,.T.);
#40789=ORIENTED_EDGE('',*,*,#27668,.F.);
#40790=ORIENTED_EDGE('',*,*,#27669,.F.);
#40791=ORIENTED_EDGE('',*,*,#27371,.T.);
#40792=ORIENTED_EDGE('',*,*,#27670,.F.);
#40793=ORIENTED_EDGE('',*,*,#27671,.F.);
#40794=ORIENTED_EDGE('',*,*,#27375,.T.);
#40795=ORIENTED_EDGE('',*,*,#27672,.F.);
#40796=ORIENTED_EDGE('',*,*,#27673,.F.);
#40797=ORIENTED_EDGE('',*,*,#27379,.T.);
#40798=ORIENTED_EDGE('',*,*,#27674,.F.);
#40799=ORIENTED_EDGE('',*,*,#27675,.F.);
#40800=ORIENTED_EDGE('',*,*,#27383,.T.);
#40801=ORIENTED_EDGE('',*,*,#27676,.F.);
#40802=ORIENTED_EDGE('',*,*,#27677,.F.);
#40803=ORIENTED_EDGE('',*,*,#27387,.T.);
#40804=ORIENTED_EDGE('',*,*,#27678,.F.);
#40805=ORIENTED_EDGE('',*,*,#27679,.F.);
#40806=ORIENTED_EDGE('',*,*,#27391,.T.);
#40807=ORIENTED_EDGE('',*,*,#27680,.F.);
#40808=ORIENTED_EDGE('',*,*,#27681,.F.);
#40809=ORIENTED_EDGE('',*,*,#27395,.T.);
#40810=ORIENTED_EDGE('',*,*,#27682,.F.);
#40811=ORIENTED_EDGE('',*,*,#27683,.F.);
#40812=ORIENTED_EDGE('',*,*,#27399,.T.);
#40813=ORIENTED_EDGE('',*,*,#27684,.F.);
#40814=ORIENTED_EDGE('',*,*,#27685,.F.);
#40815=ORIENTED_EDGE('',*,*,#27403,.T.);
#40816=ORIENTED_EDGE('',*,*,#27686,.F.);
#40817=ORIENTED_EDGE('',*,*,#27687,.F.);
#40818=ORIENTED_EDGE('',*,*,#27407,.T.);
#40819=ORIENTED_EDGE('',*,*,#27688,.F.);
#40820=ORIENTED_EDGE('',*,*,#27689,.F.);
#40821=ORIENTED_EDGE('',*,*,#27411,.T.);
#40822=ORIENTED_EDGE('',*,*,#27690,.F.);
#40823=ORIENTED_EDGE('',*,*,#27691,.F.);
#40824=ORIENTED_EDGE('',*,*,#27415,.T.);
#40825=ORIENTED_EDGE('',*,*,#27692,.F.);
#40826=ORIENTED_EDGE('',*,*,#27693,.F.);
#40827=ORIENTED_EDGE('',*,*,#27419,.T.);
#40828=ORIENTED_EDGE('',*,*,#27694,.F.);
#40829=ORIENTED_EDGE('',*,*,#27695,.F.);
#40830=ORIENTED_EDGE('',*,*,#27423,.T.);
#40831=ORIENTED_EDGE('',*,*,#27696,.F.);
#40832=ORIENTED_EDGE('',*,*,#27697,.F.);
#40833=ORIENTED_EDGE('',*,*,#27439,.T.);
#40834=ORIENTED_EDGE('',*,*,#27698,.F.);
#40835=ORIENTED_EDGE('',*,*,#27699,.F.);
#40836=ORIENTED_EDGE('',*,*,#27433,.T.);
#40837=ORIENTED_EDGE('',*,*,#27700,.F.);
#40838=ORIENTED_EDGE('',*,*,#27701,.F.);
#40839=ORIENTED_EDGE('',*,*,#27429,.T.);
#40840=ORIENTED_EDGE('',*,*,#27702,.F.);
#40841=ORIENTED_EDGE('',*,*,#27703,.F.);
#40842=ORIENTED_EDGE('',*,*,#27425,.T.);
#40843=ORIENTED_EDGE('',*,*,#27704,.F.);
#40844=ORIENTED_EDGE('',*,*,#27705,.F.);
#40845=ORIENTED_EDGE('',*,*,#27443,.T.);
#40846=ORIENTED_EDGE('',*,*,#27706,.F.);
#40847=ORIENTED_EDGE('',*,*,#27707,.F.);
#40848=ORIENTED_EDGE('',*,*,#27447,.T.);
#40849=ORIENTED_EDGE('',*,*,#27708,.F.);
#40850=ORIENTED_EDGE('',*,*,#27709,.F.);
#40851=ORIENTED_EDGE('',*,*,#27451,.T.);
#40852=ORIENTED_EDGE('',*,*,#27710,.F.);
#40853=ORIENTED_EDGE('',*,*,#27711,.F.);
#40854=ORIENTED_EDGE('',*,*,#27455,.T.);
#40855=ORIENTED_EDGE('',*,*,#27712,.F.);
#40856=ORIENTED_EDGE('',*,*,#27713,.F.);
#40857=ORIENTED_EDGE('',*,*,#27459,.T.);
#40858=ORIENTED_EDGE('',*,*,#27714,.F.);
#40859=ORIENTED_EDGE('',*,*,#27715,.F.);
#40860=ORIENTED_EDGE('',*,*,#27463,.T.);
#40861=ORIENTED_EDGE('',*,*,#27716,.F.);
#40862=ORIENTED_EDGE('',*,*,#27717,.F.);
#40863=ORIENTED_EDGE('',*,*,#27467,.T.);
#40864=ORIENTED_EDGE('',*,*,#27718,.F.);
#40865=ORIENTED_EDGE('',*,*,#27719,.F.);
#40866=ORIENTED_EDGE('',*,*,#27471,.T.);
#40867=ORIENTED_EDGE('',*,*,#27720,.F.);
#40868=ORIENTED_EDGE('',*,*,#27721,.F.);
#40869=ORIENTED_EDGE('',*,*,#27475,.T.);
#40870=ORIENTED_EDGE('',*,*,#27722,.F.);
#40871=ORIENTED_EDGE('',*,*,#27723,.F.);
#40872=ORIENTED_EDGE('',*,*,#27479,.T.);
#40873=ORIENTED_EDGE('',*,*,#27724,.F.);
#40874=ORIENTED_EDGE('',*,*,#27725,.F.);
#40875=ORIENTED_EDGE('',*,*,#27487,.T.);
#40876=ORIENTED_EDGE('',*,*,#27726,.F.);
#40877=ORIENTED_EDGE('',*,*,#27727,.F.);
#40878=ORIENTED_EDGE('',*,*,#27481,.T.);
#40879=ORIENTED_EDGE('',*,*,#27728,.F.);
#40880=ORIENTED_EDGE('',*,*,#27729,.F.);
#40881=ORIENTED_EDGE('',*,*,#27491,.T.);
#40882=ORIENTED_EDGE('',*,*,#27730,.F.);
#40883=ORIENTED_EDGE('',*,*,#27731,.F.);
#40884=ORIENTED_EDGE('',*,*,#27495,.T.);
#40885=ORIENTED_EDGE('',*,*,#27732,.F.);
#40886=ORIENTED_EDGE('',*,*,#27733,.F.);
#40887=ORIENTED_EDGE('',*,*,#27499,.T.);
#40888=ORIENTED_EDGE('',*,*,#27734,.F.);
#40889=ORIENTED_EDGE('',*,*,#27735,.F.);
#40890=ORIENTED_EDGE('',*,*,#27503,.T.);
#40891=ORIENTED_EDGE('',*,*,#27736,.F.);
#40892=ORIENTED_EDGE('',*,*,#27737,.F.);
#40893=ORIENTED_EDGE('',*,*,#27507,.T.);
#40894=ORIENTED_EDGE('',*,*,#27738,.F.);
#40895=ORIENTED_EDGE('',*,*,#27739,.F.);
#40896=ORIENTED_EDGE('',*,*,#27511,.T.);
#40897=ORIENTED_EDGE('',*,*,#27740,.F.);
#40898=ORIENTED_EDGE('',*,*,#27741,.F.);
#40899=ORIENTED_EDGE('',*,*,#27515,.T.);
#40900=ORIENTED_EDGE('',*,*,#27742,.F.);
#40901=ORIENTED_EDGE('',*,*,#27743,.F.);
#40902=ORIENTED_EDGE('',*,*,#27519,.T.);
#40903=ORIENTED_EDGE('',*,*,#27744,.F.);
#40904=ORIENTED_EDGE('',*,*,#27745,.F.);
#40905=ORIENTED_EDGE('',*,*,#27551,.T.);
#40906=ORIENTED_EDGE('',*,*,#27746,.F.);
#40907=ORIENTED_EDGE('',*,*,#27747,.F.);
#40908=ORIENTED_EDGE('',*,*,#27545,.T.);
#40909=ORIENTED_EDGE('',*,*,#27748,.F.);
#40910=ORIENTED_EDGE('',*,*,#27749,.F.);
#40911=ORIENTED_EDGE('',*,*,#27541,.T.);
#40912=ORIENTED_EDGE('',*,*,#27750,.F.);
#40913=ORIENTED_EDGE('',*,*,#27751,.F.);
#40914=ORIENTED_EDGE('',*,*,#27537,.T.);
#40915=ORIENTED_EDGE('',*,*,#27752,.F.);
#40916=ORIENTED_EDGE('',*,*,#27753,.F.);
#40917=ORIENTED_EDGE('',*,*,#27533,.T.);
#40918=ORIENTED_EDGE('',*,*,#27754,.F.);
#40919=ORIENTED_EDGE('',*,*,#27755,.F.);
#40920=ORIENTED_EDGE('',*,*,#27529,.T.);
#40921=ORIENTED_EDGE('',*,*,#27756,.F.);
#40922=ORIENTED_EDGE('',*,*,#27757,.F.);
#40923=ORIENTED_EDGE('',*,*,#27525,.T.);
#40924=ORIENTED_EDGE('',*,*,#27758,.F.);
#40925=ORIENTED_EDGE('',*,*,#27759,.F.);
#40926=ORIENTED_EDGE('',*,*,#27521,.T.);
#40927=ORIENTED_EDGE('',*,*,#27760,.F.);
#40928=ORIENTED_EDGE('',*,*,#27761,.F.);
#40929=ORIENTED_EDGE('',*,*,#27555,.T.);
#40930=ORIENTED_EDGE('',*,*,#27762,.F.);
#40931=ORIENTED_EDGE('',*,*,#27763,.F.);
#40932=ORIENTED_EDGE('',*,*,#27563,.T.);
#40933=ORIENTED_EDGE('',*,*,#27764,.F.);
#40934=ORIENTED_EDGE('',*,*,#27765,.F.);
#40935=ORIENTED_EDGE('',*,*,#27557,.T.);
#40936=ORIENTED_EDGE('',*,*,#27766,.F.);
#40937=ORIENTED_EDGE('',*,*,#27767,.F.);
#40938=ORIENTED_EDGE('',*,*,#27361,.T.);
#40939=ORIENTED_EDGE('',*,*,#27359,.F.);
#40940=ORIENTED_EDGE('',*,*,#27357,.T.);
#40941=ORIENTED_EDGE('',*,*,#27348,.F.);
#40942=ORIENTED_EDGE('',*,*,#27354,.T.);
#40943=ORIENTED_EDGE('',*,*,#27351,.F.);
#40944=ORIENTED_EDGE('',*,*,#27353,.T.);
#40945=ORIENTED_EDGE('',*,*,#27350,.T.);
#40946=ORIENTED_EDGE('',*,*,#27569,.T.);
#40947=ORIENTED_EDGE('',*,*,#27768,.T.);
#40948=ORIENTED_EDGE('',*,*,#27764,.T.);
#40949=ORIENTED_EDGE('',*,*,#27562,.F.);
#40950=ORIENTED_EDGE('',*,*,#27568,.T.);
#40951=ORIENTED_EDGE('',*,*,#27558,.T.);
#40952=ORIENTED_EDGE('',*,*,#27765,.T.);
#40953=ORIENTED_EDGE('',*,*,#27768,.F.);
#40954=ORIENTED_EDGE('',*,*,#27567,.T.);
#40955=ORIENTED_EDGE('',*,*,#27769,.T.);
#40956=ORIENTED_EDGE('',*,*,#27766,.T.);
#40957=ORIENTED_EDGE('',*,*,#27556,.F.);
#40958=ORIENTED_EDGE('',*,*,#27566,.T.);
#40959=ORIENTED_EDGE('',*,*,#27362,.T.);
#40960=ORIENTED_EDGE('',*,*,#27767,.T.);
#40961=ORIENTED_EDGE('',*,*,#27769,.F.);
#40962=ORIENTED_EDGE('',*,*,#27571,.T.);
#40963=ORIENTED_EDGE('',*,*,#27770,.T.);
#40964=ORIENTED_EDGE('',*,*,#27762,.T.);
#40965=ORIENTED_EDGE('',*,*,#27554,.F.);
#40966=ORIENTED_EDGE('',*,*,#27570,.T.);
#40967=ORIENTED_EDGE('',*,*,#27560,.T.);
#40968=ORIENTED_EDGE('',*,*,#27763,.T.);
#40969=ORIENTED_EDGE('',*,*,#27770,.F.);
#40970=ORIENTED_EDGE('',*,*,#27587,.T.);
#40971=ORIENTED_EDGE('',*,*,#27771,.T.);
#40972=ORIENTED_EDGE('',*,*,#27746,.T.);
#40973=ORIENTED_EDGE('',*,*,#27550,.F.);
#40974=ORIENTED_EDGE('',*,*,#27586,.T.);
#40975=ORIENTED_EDGE('',*,*,#27546,.T.);
#40976=ORIENTED_EDGE('',*,*,#27747,.T.);
#40977=ORIENTED_EDGE('',*,*,#27771,.F.);
#40978=ORIENTED_EDGE('',*,*,#27585,.T.);
#40979=ORIENTED_EDGE('',*,*,#27772,.T.);
#40980=ORIENTED_EDGE('',*,*,#27748,.T.);
#40981=ORIENTED_EDGE('',*,*,#27544,.F.);
#40982=ORIENTED_EDGE('',*,*,#27584,.T.);
#40983=ORIENTED_EDGE('',*,*,#27542,.T.);
#40984=ORIENTED_EDGE('',*,*,#27749,.T.);
#40985=ORIENTED_EDGE('',*,*,#27772,.F.);
#40986=ORIENTED_EDGE('',*,*,#27583,.T.);
#40987=ORIENTED_EDGE('',*,*,#27773,.T.);
#40988=ORIENTED_EDGE('',*,*,#27750,.T.);
#40989=ORIENTED_EDGE('',*,*,#27540,.F.);
#40990=ORIENTED_EDGE('',*,*,#27582,.T.);
#40991=ORIENTED_EDGE('',*,*,#27538,.T.);
#40992=ORIENTED_EDGE('',*,*,#27751,.T.);
#40993=ORIENTED_EDGE('',*,*,#27773,.F.);
#40994=ORIENTED_EDGE('',*,*,#27581,.T.);
#40995=ORIENTED_EDGE('',*,*,#27774,.T.);
#40996=ORIENTED_EDGE('',*,*,#27752,.T.);
#40997=ORIENTED_EDGE('',*,*,#27536,.F.);
#40998=ORIENTED_EDGE('',*,*,#27580,.T.);
#40999=ORIENTED_EDGE('',*,*,#27534,.T.);
#41000=ORIENTED_EDGE('',*,*,#27753,.T.);
#41001=ORIENTED_EDGE('',*,*,#27774,.F.);
#41002=ORIENTED_EDGE('',*,*,#27579,.T.);
#41003=ORIENTED_EDGE('',*,*,#27775,.T.);
#41004=ORIENTED_EDGE('',*,*,#27754,.T.);
#41005=ORIENTED_EDGE('',*,*,#27532,.F.);
#41006=ORIENTED_EDGE('',*,*,#27578,.T.);
#41007=ORIENTED_EDGE('',*,*,#27530,.T.);
#41008=ORIENTED_EDGE('',*,*,#27755,.T.);
#41009=ORIENTED_EDGE('',*,*,#27775,.F.);
#41010=ORIENTED_EDGE('',*,*,#27577,.T.);
#41011=ORIENTED_EDGE('',*,*,#27776,.T.);
#41012=ORIENTED_EDGE('',*,*,#27756,.T.);
#41013=ORIENTED_EDGE('',*,*,#27528,.F.);
#41014=ORIENTED_EDGE('',*,*,#27576,.T.);
#41015=ORIENTED_EDGE('',*,*,#27526,.T.);
#41016=ORIENTED_EDGE('',*,*,#27757,.T.);
#41017=ORIENTED_EDGE('',*,*,#27776,.F.);
#41018=ORIENTED_EDGE('',*,*,#27575,.T.);
#41019=ORIENTED_EDGE('',*,*,#27777,.T.);
#41020=ORIENTED_EDGE('',*,*,#27758,.T.);
#41021=ORIENTED_EDGE('',*,*,#27524,.F.);
#41022=ORIENTED_EDGE('',*,*,#27574,.T.);
#41023=ORIENTED_EDGE('',*,*,#27522,.T.);
#41024=ORIENTED_EDGE('',*,*,#27759,.T.);
#41025=ORIENTED_EDGE('',*,*,#27777,.F.);
#41026=ORIENTED_EDGE('',*,*,#27573,.T.);
#41027=ORIENTED_EDGE('',*,*,#27778,.T.);
#41028=ORIENTED_EDGE('',*,*,#27760,.T.);
#41029=ORIENTED_EDGE('',*,*,#27520,.F.);
#41030=ORIENTED_EDGE('',*,*,#27572,.T.);
#41031=ORIENTED_EDGE('',*,*,#27552,.T.);
#41032=ORIENTED_EDGE('',*,*,#27761,.T.);
#41033=ORIENTED_EDGE('',*,*,#27778,.F.);
#41034=ORIENTED_EDGE('',*,*,#27589,.T.);
#41035=ORIENTED_EDGE('',*,*,#27779,.T.);
#41036=ORIENTED_EDGE('',*,*,#27744,.T.);
#41037=ORIENTED_EDGE('',*,*,#27518,.F.);
#41038=ORIENTED_EDGE('',*,*,#27588,.T.);
#41039=ORIENTED_EDGE('',*,*,#27548,.T.);
#41040=ORIENTED_EDGE('',*,*,#27745,.T.);
#41041=ORIENTED_EDGE('',*,*,#27779,.F.);
#41042=ORIENTED_EDGE('',*,*,#27591,.T.);
#41043=ORIENTED_EDGE('',*,*,#27780,.T.);
#41044=ORIENTED_EDGE('',*,*,#27742,.T.);
#41045=ORIENTED_EDGE('',*,*,#27514,.F.);
#41046=ORIENTED_EDGE('',*,*,#27590,.T.);
#41047=ORIENTED_EDGE('',*,*,#27516,.T.);
#41048=ORIENTED_EDGE('',*,*,#27743,.T.);
#41049=ORIENTED_EDGE('',*,*,#27780,.F.);
#41050=ORIENTED_EDGE('',*,*,#27593,.T.);
#41051=ORIENTED_EDGE('',*,*,#27781,.T.);
#41052=ORIENTED_EDGE('',*,*,#27740,.T.);
#41053=ORIENTED_EDGE('',*,*,#27510,.F.);
#41054=ORIENTED_EDGE('',*,*,#27592,.T.);
#41055=ORIENTED_EDGE('',*,*,#27512,.T.);
#41056=ORIENTED_EDGE('',*,*,#27741,.T.);
#41057=ORIENTED_EDGE('',*,*,#27781,.F.);
#41058=ORIENTED_EDGE('',*,*,#27595,.T.);
#41059=ORIENTED_EDGE('',*,*,#27782,.T.);
#41060=ORIENTED_EDGE('',*,*,#27738,.T.);
#41061=ORIENTED_EDGE('',*,*,#27506,.F.);
#41062=ORIENTED_EDGE('',*,*,#27594,.T.);
#41063=ORIENTED_EDGE('',*,*,#27508,.T.);
#41064=ORIENTED_EDGE('',*,*,#27739,.T.);
#41065=ORIENTED_EDGE('',*,*,#27782,.F.);
#41066=ORIENTED_EDGE('',*,*,#27597,.T.);
#41067=ORIENTED_EDGE('',*,*,#27783,.T.);
#41068=ORIENTED_EDGE('',*,*,#27736,.T.);
#41069=ORIENTED_EDGE('',*,*,#27502,.F.);
#41070=ORIENTED_EDGE('',*,*,#27596,.T.);
#41071=ORIENTED_EDGE('',*,*,#27504,.T.);
#41072=ORIENTED_EDGE('',*,*,#27737,.T.);
#41073=ORIENTED_EDGE('',*,*,#27783,.F.);
#41074=ORIENTED_EDGE('',*,*,#27599,.T.);
#41075=ORIENTED_EDGE('',*,*,#27784,.T.);
#41076=ORIENTED_EDGE('',*,*,#27734,.T.);
#41077=ORIENTED_EDGE('',*,*,#27498,.F.);
#41078=ORIENTED_EDGE('',*,*,#27598,.T.);
#41079=ORIENTED_EDGE('',*,*,#27500,.T.);
#41080=ORIENTED_EDGE('',*,*,#27735,.T.);
#41081=ORIENTED_EDGE('',*,*,#27784,.F.);
#41082=ORIENTED_EDGE('',*,*,#27601,.T.);
#41083=ORIENTED_EDGE('',*,*,#27785,.T.);
#41084=ORIENTED_EDGE('',*,*,#27732,.T.);
#41085=ORIENTED_EDGE('',*,*,#27494,.F.);
#41086=ORIENTED_EDGE('',*,*,#27600,.T.);
#41087=ORIENTED_EDGE('',*,*,#27496,.T.);
#41088=ORIENTED_EDGE('',*,*,#27733,.T.);
#41089=ORIENTED_EDGE('',*,*,#27785,.F.);
#41090=ORIENTED_EDGE('',*,*,#27603,.T.);
#41091=ORIENTED_EDGE('',*,*,#27786,.T.);
#41092=ORIENTED_EDGE('',*,*,#27730,.T.);
#41093=ORIENTED_EDGE('',*,*,#27490,.F.);
#41094=ORIENTED_EDGE('',*,*,#27602,.T.);
#41095=ORIENTED_EDGE('',*,*,#27492,.T.);
#41096=ORIENTED_EDGE('',*,*,#27731,.T.);
#41097=ORIENTED_EDGE('',*,*,#27786,.F.);
#41098=ORIENTED_EDGE('',*,*,#27607,.T.);
#41099=ORIENTED_EDGE('',*,*,#27787,.T.);
#41100=ORIENTED_EDGE('',*,*,#27726,.T.);
#41101=ORIENTED_EDGE('',*,*,#27486,.F.);
#41102=ORIENTED_EDGE('',*,*,#27606,.T.);
#41103=ORIENTED_EDGE('',*,*,#27482,.T.);
#41104=ORIENTED_EDGE('',*,*,#27727,.T.);
#41105=ORIENTED_EDGE('',*,*,#27787,.F.);
#41106=ORIENTED_EDGE('',*,*,#27605,.T.);
#41107=ORIENTED_EDGE('',*,*,#27788,.T.);
#41108=ORIENTED_EDGE('',*,*,#27728,.T.);
#41109=ORIENTED_EDGE('',*,*,#27480,.F.);
#41110=ORIENTED_EDGE('',*,*,#27604,.T.);
#41111=ORIENTED_EDGE('',*,*,#27488,.T.);
#41112=ORIENTED_EDGE('',*,*,#27729,.T.);
#41113=ORIENTED_EDGE('',*,*,#27788,.F.);
#41114=ORIENTED_EDGE('',*,*,#27609,.T.);
#41115=ORIENTED_EDGE('',*,*,#27789,.T.);
#41116=ORIENTED_EDGE('',*,*,#27724,.T.);
#41117=ORIENTED_EDGE('',*,*,#27478,.F.);
#41118=ORIENTED_EDGE('',*,*,#27608,.T.);
#41119=ORIENTED_EDGE('',*,*,#27484,.T.);
#41120=ORIENTED_EDGE('',*,*,#27725,.T.);
#41121=ORIENTED_EDGE('',*,*,#27789,.F.);
#41122=ORIENTED_EDGE('',*,*,#27611,.T.);
#41123=ORIENTED_EDGE('',*,*,#27790,.T.);
#41124=ORIENTED_EDGE('',*,*,#27722,.T.);
#41125=ORIENTED_EDGE('',*,*,#27474,.F.);
#41126=ORIENTED_EDGE('',*,*,#27610,.T.);
#41127=ORIENTED_EDGE('',*,*,#27476,.T.);
#41128=ORIENTED_EDGE('',*,*,#27723,.T.);
#41129=ORIENTED_EDGE('',*,*,#27790,.F.);
#41130=ORIENTED_EDGE('',*,*,#27613,.T.);
#41131=ORIENTED_EDGE('',*,*,#27791,.T.);
#41132=ORIENTED_EDGE('',*,*,#27720,.T.);
#41133=ORIENTED_EDGE('',*,*,#27470,.F.);
#41134=ORIENTED_EDGE('',*,*,#27612,.T.);
#41135=ORIENTED_EDGE('',*,*,#27472,.T.);
#41136=ORIENTED_EDGE('',*,*,#27721,.T.);
#41137=ORIENTED_EDGE('',*,*,#27791,.F.);
#41138=ORIENTED_EDGE('',*,*,#27615,.T.);
#41139=ORIENTED_EDGE('',*,*,#27792,.T.);
#41140=ORIENTED_EDGE('',*,*,#27718,.T.);
#41141=ORIENTED_EDGE('',*,*,#27466,.F.);
#41142=ORIENTED_EDGE('',*,*,#27614,.T.);
#41143=ORIENTED_EDGE('',*,*,#27468,.T.);
#41144=ORIENTED_EDGE('',*,*,#27719,.T.);
#41145=ORIENTED_EDGE('',*,*,#27792,.F.);
#41146=ORIENTED_EDGE('',*,*,#27617,.T.);
#41147=ORIENTED_EDGE('',*,*,#27793,.T.);
#41148=ORIENTED_EDGE('',*,*,#27716,.T.);
#41149=ORIENTED_EDGE('',*,*,#27462,.F.);
#41150=ORIENTED_EDGE('',*,*,#27616,.T.);
#41151=ORIENTED_EDGE('',*,*,#27464,.T.);
#41152=ORIENTED_EDGE('',*,*,#27717,.T.);
#41153=ORIENTED_EDGE('',*,*,#27793,.F.);
#41154=ORIENTED_EDGE('',*,*,#27619,.T.);
#41155=ORIENTED_EDGE('',*,*,#27794,.T.);
#41156=ORIENTED_EDGE('',*,*,#27714,.T.);
#41157=ORIENTED_EDGE('',*,*,#27458,.F.);
#41158=ORIENTED_EDGE('',*,*,#27618,.T.);
#41159=ORIENTED_EDGE('',*,*,#27460,.T.);
#41160=ORIENTED_EDGE('',*,*,#27715,.T.);
#41161=ORIENTED_EDGE('',*,*,#27794,.F.);
#41162=ORIENTED_EDGE('',*,*,#27621,.T.);
#41163=ORIENTED_EDGE('',*,*,#27795,.T.);
#41164=ORIENTED_EDGE('',*,*,#27712,.T.);
#41165=ORIENTED_EDGE('',*,*,#27454,.F.);
#41166=ORIENTED_EDGE('',*,*,#27620,.T.);
#41167=ORIENTED_EDGE('',*,*,#27456,.T.);
#41168=ORIENTED_EDGE('',*,*,#27713,.T.);
#41169=ORIENTED_EDGE('',*,*,#27795,.F.);
#41170=ORIENTED_EDGE('',*,*,#27623,.T.);
#41171=ORIENTED_EDGE('',*,*,#27796,.T.);
#41172=ORIENTED_EDGE('',*,*,#27710,.T.);
#41173=ORIENTED_EDGE('',*,*,#27450,.F.);
#41174=ORIENTED_EDGE('',*,*,#27622,.T.);
#41175=ORIENTED_EDGE('',*,*,#27452,.T.);
#41176=ORIENTED_EDGE('',*,*,#27711,.T.);
#41177=ORIENTED_EDGE('',*,*,#27796,.F.);
#41178=ORIENTED_EDGE('',*,*,#27625,.T.);
#41179=ORIENTED_EDGE('',*,*,#27797,.T.);
#41180=ORIENTED_EDGE('',*,*,#27708,.T.);
#41181=ORIENTED_EDGE('',*,*,#27446,.F.);
#41182=ORIENTED_EDGE('',*,*,#27624,.T.);
#41183=ORIENTED_EDGE('',*,*,#27448,.T.);
#41184=ORIENTED_EDGE('',*,*,#27709,.T.);
#41185=ORIENTED_EDGE('',*,*,#27797,.F.);
#41186=ORIENTED_EDGE('',*,*,#27627,.T.);
#41187=ORIENTED_EDGE('',*,*,#27798,.T.);
#41188=ORIENTED_EDGE('',*,*,#27706,.T.);
#41189=ORIENTED_EDGE('',*,*,#27442,.F.);
#41190=ORIENTED_EDGE('',*,*,#27626,.T.);
#41191=ORIENTED_EDGE('',*,*,#27444,.T.);
#41192=ORIENTED_EDGE('',*,*,#27707,.T.);
#41193=ORIENTED_EDGE('',*,*,#27798,.F.);
#41194=ORIENTED_EDGE('',*,*,#27635,.T.);
#41195=ORIENTED_EDGE('',*,*,#27799,.T.);
#41196=ORIENTED_EDGE('',*,*,#27698,.T.);
#41197=ORIENTED_EDGE('',*,*,#27438,.F.);
#41198=ORIENTED_EDGE('',*,*,#27634,.T.);
#41199=ORIENTED_EDGE('',*,*,#27434,.T.);
#41200=ORIENTED_EDGE('',*,*,#27699,.T.);
#41201=ORIENTED_EDGE('',*,*,#27799,.F.);
#41202=ORIENTED_EDGE('',*,*,#27633,.T.);
#41203=ORIENTED_EDGE('',*,*,#27800,.T.);
#41204=ORIENTED_EDGE('',*,*,#27700,.T.);
#41205=ORIENTED_EDGE('',*,*,#27432,.F.);
#41206=ORIENTED_EDGE('',*,*,#27632,.T.);
#41207=ORIENTED_EDGE('',*,*,#27430,.T.);
#41208=ORIENTED_EDGE('',*,*,#27701,.T.);
#41209=ORIENTED_EDGE('',*,*,#27800,.F.);
#41210=ORIENTED_EDGE('',*,*,#27631,.T.);
#41211=ORIENTED_EDGE('',*,*,#27801,.T.);
#41212=ORIENTED_EDGE('',*,*,#27702,.T.);
#41213=ORIENTED_EDGE('',*,*,#27428,.F.);
#41214=ORIENTED_EDGE('',*,*,#27630,.T.);
#41215=ORIENTED_EDGE('',*,*,#27426,.T.);
#41216=ORIENTED_EDGE('',*,*,#27703,.T.);
#41217=ORIENTED_EDGE('',*,*,#27801,.F.);
#41218=ORIENTED_EDGE('',*,*,#27629,.T.);
#41219=ORIENTED_EDGE('',*,*,#27802,.T.);
#41220=ORIENTED_EDGE('',*,*,#27704,.T.);
#41221=ORIENTED_EDGE('',*,*,#27424,.F.);
#41222=ORIENTED_EDGE('',*,*,#27628,.T.);
#41223=ORIENTED_EDGE('',*,*,#27440,.T.);
#41224=ORIENTED_EDGE('',*,*,#27705,.T.);
#41225=ORIENTED_EDGE('',*,*,#27802,.F.);
#41226=ORIENTED_EDGE('',*,*,#27637,.T.);
#41227=ORIENTED_EDGE('',*,*,#27803,.T.);
#41228=ORIENTED_EDGE('',*,*,#27696,.T.);
#41229=ORIENTED_EDGE('',*,*,#27422,.F.);
#41230=ORIENTED_EDGE('',*,*,#27636,.T.);
#41231=ORIENTED_EDGE('',*,*,#27436,.T.);
#41232=ORIENTED_EDGE('',*,*,#27697,.T.);
#41233=ORIENTED_EDGE('',*,*,#27803,.F.);
#41234=ORIENTED_EDGE('',*,*,#27639,.T.);
#41235=ORIENTED_EDGE('',*,*,#27804,.T.);
#41236=ORIENTED_EDGE('',*,*,#27694,.T.);
#41237=ORIENTED_EDGE('',*,*,#27418,.F.);
#41238=ORIENTED_EDGE('',*,*,#27638,.T.);
#41239=ORIENTED_EDGE('',*,*,#27420,.T.);
#41240=ORIENTED_EDGE('',*,*,#27695,.T.);
#41241=ORIENTED_EDGE('',*,*,#27804,.F.);
#41242=ORIENTED_EDGE('',*,*,#27641,.T.);
#41243=ORIENTED_EDGE('',*,*,#27805,.T.);
#41244=ORIENTED_EDGE('',*,*,#27692,.T.);
#41245=ORIENTED_EDGE('',*,*,#27414,.F.);
#41246=ORIENTED_EDGE('',*,*,#27640,.T.);
#41247=ORIENTED_EDGE('',*,*,#27416,.T.);
#41248=ORIENTED_EDGE('',*,*,#27693,.T.);
#41249=ORIENTED_EDGE('',*,*,#27805,.F.);
#41250=ORIENTED_EDGE('',*,*,#27643,.T.);
#41251=ORIENTED_EDGE('',*,*,#27806,.T.);
#41252=ORIENTED_EDGE('',*,*,#27690,.T.);
#41253=ORIENTED_EDGE('',*,*,#27410,.F.);
#41254=ORIENTED_EDGE('',*,*,#27642,.T.);
#41255=ORIENTED_EDGE('',*,*,#27412,.T.);
#41256=ORIENTED_EDGE('',*,*,#27691,.T.);
#41257=ORIENTED_EDGE('',*,*,#27806,.F.);
#41258=ORIENTED_EDGE('',*,*,#27645,.T.);
#41259=ORIENTED_EDGE('',*,*,#27807,.T.);
#41260=ORIENTED_EDGE('',*,*,#27688,.T.);
#41261=ORIENTED_EDGE('',*,*,#27406,.F.);
#41262=ORIENTED_EDGE('',*,*,#27644,.T.);
#41263=ORIENTED_EDGE('',*,*,#27408,.T.);
#41264=ORIENTED_EDGE('',*,*,#27689,.T.);
#41265=ORIENTED_EDGE('',*,*,#27807,.F.);
#41266=ORIENTED_EDGE('',*,*,#27647,.T.);
#41267=ORIENTED_EDGE('',*,*,#27808,.T.);
#41268=ORIENTED_EDGE('',*,*,#27686,.T.);
#41269=ORIENTED_EDGE('',*,*,#27402,.F.);
#41270=ORIENTED_EDGE('',*,*,#27646,.T.);
#41271=ORIENTED_EDGE('',*,*,#27404,.T.);
#41272=ORIENTED_EDGE('',*,*,#27687,.T.);
#41273=ORIENTED_EDGE('',*,*,#27808,.F.);
#41274=ORIENTED_EDGE('',*,*,#27649,.T.);
#41275=ORIENTED_EDGE('',*,*,#27809,.T.);
#41276=ORIENTED_EDGE('',*,*,#27684,.T.);
#41277=ORIENTED_EDGE('',*,*,#27398,.F.);
#41278=ORIENTED_EDGE('',*,*,#27648,.T.);
#41279=ORIENTED_EDGE('',*,*,#27400,.T.);
#41280=ORIENTED_EDGE('',*,*,#27685,.T.);
#41281=ORIENTED_EDGE('',*,*,#27809,.F.);
#41282=ORIENTED_EDGE('',*,*,#27651,.T.);
#41283=ORIENTED_EDGE('',*,*,#27810,.T.);
#41284=ORIENTED_EDGE('',*,*,#27682,.T.);
#41285=ORIENTED_EDGE('',*,*,#27394,.F.);
#41286=ORIENTED_EDGE('',*,*,#27650,.T.);
#41287=ORIENTED_EDGE('',*,*,#27396,.T.);
#41288=ORIENTED_EDGE('',*,*,#27683,.T.);
#41289=ORIENTED_EDGE('',*,*,#27810,.F.);
#41290=ORIENTED_EDGE('',*,*,#27653,.T.);
#41291=ORIENTED_EDGE('',*,*,#27811,.T.);
#41292=ORIENTED_EDGE('',*,*,#27680,.T.);
#41293=ORIENTED_EDGE('',*,*,#27390,.F.);
#41294=ORIENTED_EDGE('',*,*,#27652,.T.);
#41295=ORIENTED_EDGE('',*,*,#27392,.T.);
#41296=ORIENTED_EDGE('',*,*,#27681,.T.);
#41297=ORIENTED_EDGE('',*,*,#27811,.F.);
#41298=ORIENTED_EDGE('',*,*,#27655,.T.);
#41299=ORIENTED_EDGE('',*,*,#27812,.T.);
#41300=ORIENTED_EDGE('',*,*,#27678,.T.);
#41301=ORIENTED_EDGE('',*,*,#27386,.F.);
#41302=ORIENTED_EDGE('',*,*,#27654,.T.);
#41303=ORIENTED_EDGE('',*,*,#27388,.T.);
#41304=ORIENTED_EDGE('',*,*,#27679,.T.);
#41305=ORIENTED_EDGE('',*,*,#27812,.F.);
#41306=ORIENTED_EDGE('',*,*,#27657,.T.);
#41307=ORIENTED_EDGE('',*,*,#27813,.T.);
#41308=ORIENTED_EDGE('',*,*,#27676,.T.);
#41309=ORIENTED_EDGE('',*,*,#27382,.F.);
#41310=ORIENTED_EDGE('',*,*,#27656,.T.);
#41311=ORIENTED_EDGE('',*,*,#27384,.T.);
#41312=ORIENTED_EDGE('',*,*,#27677,.T.);
#41313=ORIENTED_EDGE('',*,*,#27813,.F.);
#41314=ORIENTED_EDGE('',*,*,#27659,.T.);
#41315=ORIENTED_EDGE('',*,*,#27814,.T.);
#41316=ORIENTED_EDGE('',*,*,#27674,.T.);
#41317=ORIENTED_EDGE('',*,*,#27378,.F.);
#41318=ORIENTED_EDGE('',*,*,#27658,.T.);
#41319=ORIENTED_EDGE('',*,*,#27380,.T.);
#41320=ORIENTED_EDGE('',*,*,#27675,.T.);
#41321=ORIENTED_EDGE('',*,*,#27814,.F.);
#41322=ORIENTED_EDGE('',*,*,#27661,.T.);
#41323=ORIENTED_EDGE('',*,*,#27815,.T.);
#41324=ORIENTED_EDGE('',*,*,#27672,.T.);
#41325=ORIENTED_EDGE('',*,*,#27374,.F.);
#41326=ORIENTED_EDGE('',*,*,#27660,.T.);
#41327=ORIENTED_EDGE('',*,*,#27376,.T.);
#41328=ORIENTED_EDGE('',*,*,#27673,.T.);
#41329=ORIENTED_EDGE('',*,*,#27815,.F.);
#41330=ORIENTED_EDGE('',*,*,#27663,.T.);
#41331=ORIENTED_EDGE('',*,*,#27816,.T.);
#41332=ORIENTED_EDGE('',*,*,#27670,.T.);
#41333=ORIENTED_EDGE('',*,*,#27370,.F.);
#41334=ORIENTED_EDGE('',*,*,#27662,.T.);
#41335=ORIENTED_EDGE('',*,*,#27372,.T.);
#41336=ORIENTED_EDGE('',*,*,#27671,.T.);
#41337=ORIENTED_EDGE('',*,*,#27816,.F.);
#41338=ORIENTED_EDGE('',*,*,#27665,.T.);
#41339=ORIENTED_EDGE('',*,*,#27817,.T.);
#41340=ORIENTED_EDGE('',*,*,#27668,.T.);
#41341=ORIENTED_EDGE('',*,*,#27366,.F.);
#41342=ORIENTED_EDGE('',*,*,#27664,.T.);
#41343=ORIENTED_EDGE('',*,*,#27368,.T.);
#41344=ORIENTED_EDGE('',*,*,#27669,.T.);
#41345=ORIENTED_EDGE('',*,*,#27817,.F.);
#41346=ORIENTED_EDGE('',*,*,#27565,.T.);
#41347=ORIENTED_EDGE('',*,*,#27818,.T.);
#41348=ORIENTED_EDGE('',*,*,#27666,.T.);
#41349=ORIENTED_EDGE('',*,*,#27360,.F.);
#41350=ORIENTED_EDGE('',*,*,#27564,.T.);
#41351=ORIENTED_EDGE('',*,*,#27364,.T.);
#41352=ORIENTED_EDGE('',*,*,#27667,.T.);
#41353=ORIENTED_EDGE('',*,*,#27818,.F.);
#42525=CYLINDRICAL_SURFACE('',#49900,0.004);
#42526=CYLINDRICAL_SURFACE('',#49903,0.005825);
#42527=CYLINDRICAL_SURFACE('',#49906,0.010875);
#42528=CYLINDRICAL_SURFACE('',#49909,0.010875);
#42529=CYLINDRICAL_SURFACE('',#49912,0.0135);
#42530=CYLINDRICAL_SURFACE('',#49915,0.0135);
#42531=CYLINDRICAL_SURFACE('',#49918,0.0135);
#42532=CYLINDRICAL_SURFACE('',#49921,0.0135);
#42533=CYLINDRICAL_SURFACE('',#49924,0.0135);
#42534=CYLINDRICAL_SURFACE('',#49927,0.0135);
#42535=CYLINDRICAL_SURFACE('',#49930,0.0135);
#42536=CYLINDRICAL_SURFACE('',#49933,0.0135);
#42537=CYLINDRICAL_SURFACE('',#49936,0.0135);
#42538=CYLINDRICAL_SURFACE('',#49939,0.0135);
#42539=CYLINDRICAL_SURFACE('',#49942,0.0135);
#42540=CYLINDRICAL_SURFACE('',#49945,0.0135);
#42541=CYLINDRICAL_SURFACE('',#49948,0.0135);
#42542=CYLINDRICAL_SURFACE('',#49951,0.0135);
#42543=CYLINDRICAL_SURFACE('',#49954,0.0135);
#42544=CYLINDRICAL_SURFACE('',#49957,0.0135);
#42545=CYLINDRICAL_SURFACE('',#49960,0.0135);
#42546=CYLINDRICAL_SURFACE('',#49963,0.0135);
#42547=CYLINDRICAL_SURFACE('',#49966,0.0135);
#42548=CYLINDRICAL_SURFACE('',#49969,0.0135);
#42549=CYLINDRICAL_SURFACE('',#49972,0.0135);
#42550=CYLINDRICAL_SURFACE('',#49975,0.0135);
#42551=CYLINDRICAL_SURFACE('',#49978,0.0135);
#42552=CYLINDRICAL_SURFACE('',#49981,0.0135);
#42553=CYLINDRICAL_SURFACE('',#49984,0.0135);
#42554=CYLINDRICAL_SURFACE('',#49987,0.0135);
#42555=CYLINDRICAL_SURFACE('',#49990,0.0135);
#42556=CYLINDRICAL_SURFACE('',#49993,0.0135);
#42557=CYLINDRICAL_SURFACE('',#49996,0.0135);
#42558=CYLINDRICAL_SURFACE('',#49999,0.0135);
#42559=CYLINDRICAL_SURFACE('',#50002,0.0135);
#42560=CYLINDRICAL_SURFACE('',#50005,0.0135);
#42561=CYLINDRICAL_SURFACE('',#50008,0.0135);
#42562=CYLINDRICAL_SURFACE('',#50011,0.0135);
#42563=CYLINDRICAL_SURFACE('',#50014,0.0135);
#42564=CYLINDRICAL_SURFACE('',#50017,0.0135);
#42565=CYLINDRICAL_SURFACE('',#50020,0.0135);
#42566=CYLINDRICAL_SURFACE('',#50023,0.0135);
#42567=CYLINDRICAL_SURFACE('',#50026,0.0135);
#42568=CYLINDRICAL_SURFACE('',#50029,0.0135);
#42569=CYLINDRICAL_SURFACE('',#50032,0.0135);
#42570=CYLINDRICAL_SURFACE('',#50035,0.0135);
#42571=CYLINDRICAL_SURFACE('',#50038,0.0135);
#42572=CYLINDRICAL_SURFACE('',#50041,0.0135);
#42573=CYLINDRICAL_SURFACE('',#50044,0.0135);
#42574=CYLINDRICAL_SURFACE('',#50047,0.0135);
#42575=CYLINDRICAL_SURFACE('',#50050,0.0135);
#42576=CYLINDRICAL_SURFACE('',#50053,0.0135);
#42577=CYLINDRICAL_SURFACE('',#50056,0.0135);
#42578=CYLINDRICAL_SURFACE('',#50059,0.0135);
#42579=CYLINDRICAL_SURFACE('',#50062,0.0135);
#45264=ADVANCED_FACE('',(#6409),#42525,.T.);
#45265=ADVANCED_FACE('',(#6410),#42526,.T.);
#45266=ADVANCED_FACE('',(#6411),#42527,.F.);
#45267=ADVANCED_FACE('',(#6412),#42528,.F.);
#45268=ADVANCED_FACE('',(#6413),#42529,.T.);
#45269=ADVANCED_FACE('',(#6414),#42530,.T.);
#45270=ADVANCED_FACE('',(#6415),#42531,.T.);
#45271=ADVANCED_FACE('',(#6416),#42532,.T.);
#45272=ADVANCED_FACE('',(#6417),#42533,.T.);
#45273=ADVANCED_FACE('',(#6418),#42534,.T.);
#45274=ADVANCED_FACE('',(#6419),#42535,.T.);
#45275=ADVANCED_FACE('',(#6420),#42536,.T.);
#45276=ADVANCED_FACE('',(#6421),#42537,.T.);
#45277=ADVANCED_FACE('',(#6422),#42538,.T.);
#45278=ADVANCED_FACE('',(#6423),#42539,.T.);
#45279=ADVANCED_FACE('',(#6424),#42540,.T.);
#45280=ADVANCED_FACE('',(#6425),#42541,.T.);
#45281=ADVANCED_FACE('',(#6426),#42542,.T.);
#45282=ADVANCED_FACE('',(#6427),#42543,.T.);
#45283=ADVANCED_FACE('',(#6428),#42544,.T.);
#45284=ADVANCED_FACE('',(#6429),#42545,.T.);
#45285=ADVANCED_FACE('',(#6430),#42546,.T.);
#45286=ADVANCED_FACE('',(#6431),#42547,.T.);
#45287=ADVANCED_FACE('',(#6432),#42548,.T.);
#45288=ADVANCED_FACE('',(#6433),#42549,.T.);
#45289=ADVANCED_FACE('',(#6434),#42550,.T.);
#45290=ADVANCED_FACE('',(#6435),#42551,.T.);
#45291=ADVANCED_FACE('',(#6436),#42552,.T.);
#45292=ADVANCED_FACE('',(#6437),#42553,.T.);
#45293=ADVANCED_FACE('',(#6438),#42554,.T.);
#45294=ADVANCED_FACE('',(#6439),#42555,.T.);
#45295=ADVANCED_FACE('',(#6440),#42556,.T.);
#45296=ADVANCED_FACE('',(#6441),#42557,.T.);
#45297=ADVANCED_FACE('',(#6442),#42558,.T.);
#45298=ADVANCED_FACE('',(#6443),#42559,.T.);
#45299=ADVANCED_FACE('',(#6444),#42560,.T.);
#45300=ADVANCED_FACE('',(#6445),#42561,.T.);
#45301=ADVANCED_FACE('',(#6446),#42562,.T.);
#45302=ADVANCED_FACE('',(#6447),#42563,.T.);
#45303=ADVANCED_FACE('',(#6448),#42564,.T.);
#45304=ADVANCED_FACE('',(#6449),#42565,.T.);
#45305=ADVANCED_FACE('',(#6450),#42566,.T.);
#45306=ADVANCED_FACE('',(#6451),#42567,.T.);
#45307=ADVANCED_FACE('',(#6452),#42568,.T.);
#45308=ADVANCED_FACE('',(#6453),#42569,.T.);
#45309=ADVANCED_FACE('',(#6454),#42570,.T.);
#45310=ADVANCED_FACE('',(#6455),#42571,.T.);
#45311=ADVANCED_FACE('',(#6456),#42572,.T.);
#45312=ADVANCED_FACE('',(#6457),#42573,.T.);
#45313=ADVANCED_FACE('',(#6458),#42574,.T.);
#45314=ADVANCED_FACE('',(#6459),#42575,.T.);
#45315=ADVANCED_FACE('',(#6460),#42576,.T.);
#45316=ADVANCED_FACE('',(#6461),#42577,.T.);
#45317=ADVANCED_FACE('',(#6462),#42578,.T.);
#45318=ADVANCED_FACE('',(#6463),#42579,.T.);
#45319=ADVANCED_FACE('',(#6464,#3519),#3574,.F.);
#45320=ADVANCED_FACE('',(#6465,#3520),#3575,.T.);
#45321=ADVANCED_FACE('',(#6466,#3521),#3576,.T.);
#45322=ADVANCED_FACE('',(#6467,#3522),#3577,.T.);
#45323=ADVANCED_FACE('',(#6468),#3578,.T.);
#45324=ADVANCED_FACE('',(#6469),#3579,.T.);
#45325=ADVANCED_FACE('',(#6470),#3580,.F.);
#45326=ADVANCED_FACE('',(#6471),#3581,.F.);
#45327=ADVANCED_FACE('',(#6472),#3582,.F.);
#45328=ADVANCED_FACE('',(#6473),#3583,.F.);
#45329=ADVANCED_FACE('',(#6474),#3584,.F.);
#45330=ADVANCED_FACE('',(#6475),#3585,.F.);
#45331=ADVANCED_FACE('',(#6476),#3586,.F.);
#45332=ADVANCED_FACE('',(#6477),#3587,.F.);
#45333=ADVANCED_FACE('',(#6478),#3588,.F.);
#45334=ADVANCED_FACE('',(#6479),#3589,.F.);
#45335=ADVANCED_FACE('',(#6480),#3590,.F.);
#45336=ADVANCED_FACE('',(#6481),#3591,.F.);
#45337=ADVANCED_FACE('',(#6482),#3592,.F.);
#45338=ADVANCED_FACE('',(#6483),#3593,.F.);
#45339=ADVANCED_FACE('',(#6484),#3594,.F.);
#45340=ADVANCED_FACE('',(#6485),#3595,.F.);
#45341=ADVANCED_FACE('',(#6486),#3596,.F.);
#45342=ADVANCED_FACE('',(#6487),#3597,.F.);
#45343=ADVANCED_FACE('',(#6488),#3598,.F.);
#45344=ADVANCED_FACE('',(#6489),#3599,.F.);
#45345=ADVANCED_FACE('',(#6490),#3600,.F.);
#45346=ADVANCED_FACE('',(#6491),#3601,.F.);
#45347=ADVANCED_FACE('',(#6492),#3602,.F.);
#45348=ADVANCED_FACE('',(#6493),#3603,.F.);
#45349=ADVANCED_FACE('',(#6494),#3604,.F.);
#45350=ADVANCED_FACE('',(#6495),#3605,.F.);
#45351=ADVANCED_FACE('',(#6496),#3606,.F.);
#45352=ADVANCED_FACE('',(#6497),#3607,.F.);
#45353=ADVANCED_FACE('',(#6498),#3608,.F.);
#45354=ADVANCED_FACE('',(#6499),#3609,.F.);
#45355=ADVANCED_FACE('',(#6500),#3610,.F.);
#45356=ADVANCED_FACE('',(#6501),#3611,.F.);
#45357=ADVANCED_FACE('',(#6502),#3612,.F.);
#45358=ADVANCED_FACE('',(#6503),#3613,.F.);
#45359=ADVANCED_FACE('',(#6504),#3614,.F.);
#45360=ADVANCED_FACE('',(#6505),#3615,.F.);
#45361=ADVANCED_FACE('',(#6506),#3616,.F.);
#45362=ADVANCED_FACE('',(#6507),#3617,.F.);
#45363=ADVANCED_FACE('',(#6508),#3618,.F.);
#45364=ADVANCED_FACE('',(#6509),#3619,.F.);
#45365=ADVANCED_FACE('',(#6510),#3620,.F.);
#45366=ADVANCED_FACE('',(#6511),#3621,.F.);
#45367=ADVANCED_FACE('',(#6512),#3622,.F.);
#45368=ADVANCED_FACE('',(#6513),#3623,.F.);
#45369=ADVANCED_FACE('',(#6514),#3624,.F.);
#45370=ADVANCED_FACE('',(#6515),#3625,.F.);
#45371=ADVANCED_FACE('',(#6516),#3626,.F.);
#45372=ADVANCED_FACE('',(#6517),#3627,.F.);
#45373=ADVANCED_FACE('',(#6518),#3628,.F.);
#45374=ADVANCED_FACE('',(#6519),#3629,.F.);
#45375=ADVANCED_FACE('',(#6520),#3630,.F.);
#45376=ADVANCED_FACE('',(#6521),#3631,.F.);
#45377=ADVANCED_FACE('',(#6522),#3632,.F.);
#45378=ADVANCED_FACE('',(#6523),#3633,.F.);
#45379=ADVANCED_FACE('',(#6524),#3634,.F.);
#45380=ADVANCED_FACE('',(#6525),#3635,.F.);
#45381=ADVANCED_FACE('',(#6526),#3636,.F.);
#45382=ADVANCED_FACE('',(#6527),#3637,.F.);
#45383=ADVANCED_FACE('',(#6528),#3638,.F.);
#45384=ADVANCED_FACE('',(#6529),#3639,.F.);
#45385=ADVANCED_FACE('',(#6530),#3640,.F.);
#45386=ADVANCED_FACE('',(#6531),#3641,.F.);
#45387=ADVANCED_FACE('',(#6532),#3642,.F.);
#45388=ADVANCED_FACE('',(#6533),#3643,.F.);
#45389=ADVANCED_FACE('',(#6534),#3644,.F.);
#45390=ADVANCED_FACE('',(#6535),#3645,.F.);
#45391=ADVANCED_FACE('',(#6536),#3646,.F.);
#45392=ADVANCED_FACE('',(#6537),#3647,.F.);
#45393=ADVANCED_FACE('',(#6538),#3648,.F.);
#45394=ADVANCED_FACE('',(#6539),#3649,.F.);
#45395=ADVANCED_FACE('',(#6540),#3650,.F.);
#45396=ADVANCED_FACE('',(#6541),#3651,.F.);
#45397=ADVANCED_FACE('',(#6542),#3652,.F.);
#45398=ADVANCED_FACE('',(#6543),#3653,.F.);
#45399=ADVANCED_FACE('',(#6544),#3654,.F.);
#45400=ADVANCED_FACE('',(#6545),#3655,.F.);
#45401=ADVANCED_FACE('',(#6546),#3656,.F.);
#45402=ADVANCED_FACE('',(#6547),#3657,.F.);
#45403=ADVANCED_FACE('',(#6548),#3658,.F.);
#45404=ADVANCED_FACE('',(#6549),#3659,.F.);
#45405=ADVANCED_FACE('',(#6550),#3660,.F.);
#45406=ADVANCED_FACE('',(#6551),#3661,.F.);
#45407=ADVANCED_FACE('',(#6552),#3662,.F.);
#45408=ADVANCED_FACE('',(#6553),#3663,.F.);
#45409=ADVANCED_FACE('',(#6554),#3664,.F.);
#45410=ADVANCED_FACE('',(#6555),#3665,.F.);
#45411=ADVANCED_FACE('',(#6556),#3666,.F.);
#45412=ADVANCED_FACE('',(#6557),#3667,.F.);
#45413=ADVANCED_FACE('',(#6558),#3668,.F.);
#45414=ADVANCED_FACE('',(#6559),#3669,.F.);
#45415=ADVANCED_FACE('',(#6560),#3670,.F.);
#45416=ADVANCED_FACE('',(#6561),#3671,.F.);
#45417=ADVANCED_FACE('',(#6562),#3672,.F.);
#45418=ADVANCED_FACE('',(#6563),#3673,.F.);
#45419=ADVANCED_FACE('',(#6564),#3674,.F.);
#45420=ADVANCED_FACE('',(#6565),#3675,.F.);
#45421=ADVANCED_FACE('',(#6566),#3676,.F.);
#45422=ADVANCED_FACE('',(#6567),#3677,.F.);
#45423=ADVANCED_FACE('',(#6568),#3678,.F.);
#45424=ADVANCED_FACE('',(#6569),#3679,.F.);
#45425=ADVANCED_FACE('',(#6570),#3680,.F.);
#45426=ADVANCED_FACE('',(#6571),#3681,.F.);
#45545=CLOSED_SHELL('',(#45264,#45265,#45266,#45267,#45268,#45269,#45270,
#45271,#45272,#45273,#45274,#45275,#45276,#45277,#45278,#45279,#45280,#45281,
#45282,#45283,#45284,#45285,#45286,#45287,#45288,#45289,#45290,#45291,#45292,
#45293,#45294,#45295,#45296,#45297,#45298,#45299,#45300,#45301,#45302,#45303,
#45304,#45305,#45306,#45307,#45308,#45309,#45310,#45311,#45312,#45313,#45314,
#45315,#45316,#45317,#45318,#45319,#45320,#45321,#45322,#45323,#45324,#45325,
#45326,#45327,#45328,#45329,#45330,#45331,#45332,#45333,#45334,#45335,#45336,
#45337,#45338,#45339,#45340,#45341,#45342,#45343,#45344,#45345,#45346,#45347,
#45348,#45349,#45350,#45351,#45352,#45353,#45354,#45355,#45356,#45357,#45358,
#45359,#45360,#45361,#45362,#45363,#45364,#45365,#45366,#45367,#45368,#45369,
#45370,#45371,#45372,#45373,#45374,#45375,#45376,#45377,#45378,#45379,#45380,
#45381,#45382,#45383,#45384,#45385,#45386,#45387,#45388,#45389,#45390,#45391,
#45392,#45393,#45394,#45395,#45396,#45397,#45398,#45399,#45400,#45401,#45402,
#45403,#45404,#45405,#45406,#45407,#45408,#45409,#45410,#45411,#45412,#45413,
#45414,#45415,#45416,#45417,#45418,#45419,#45420,#45421,#45422,#45423,#45424,
#45425,#45426));
#49899=AXIS2_PLACEMENT_3D('',#106261,#60263,#60264);
#49900=AXIS2_PLACEMENT_3D('',#106262,#60265,#60266);
#49901=AXIS2_PLACEMENT_3D('',#106264,#60267,#60268);
#49902=AXIS2_PLACEMENT_3D('',#106267,#60270,#60271);
#49903=AXIS2_PLACEMENT_3D('',#106268,#60272,#60273);
#49904=AXIS2_PLACEMENT_3D('',#106270,#60274,#60275);
#49905=AXIS2_PLACEMENT_3D('',#106273,#60277,#60278);
#49906=AXIS2_PLACEMENT_3D('',#106274,#60279,#60280);
#49907=AXIS2_PLACEMENT_3D('',#106276,#60281,#60282);
#49908=AXIS2_PLACEMENT_3D('',#106279,#60284,#60285);
#49909=AXIS2_PLACEMENT_3D('',#106280,#60286,#60287);
#49910=AXIS2_PLACEMENT_3D('',#106282,#60288,#60289);
#49911=AXIS2_PLACEMENT_3D('',#106285,#60291,#60292);
#49912=AXIS2_PLACEMENT_3D('',#106286,#60293,#60294);
#49913=AXIS2_PLACEMENT_3D('',#106291,#60296,#60297);
#49914=AXIS2_PLACEMENT_3D('',#106294,#60299,#60300);
#49915=AXIS2_PLACEMENT_3D('',#106295,#60301,#60302);
#49916=AXIS2_PLACEMENT_3D('',#106300,#60304,#60305);
#49917=AXIS2_PLACEMENT_3D('',#106303,#60307,#60308);
#49918=AXIS2_PLACEMENT_3D('',#106304,#60309,#60310);
#49919=AXIS2_PLACEMENT_3D('',#106309,#60312,#60313);
#49920=AXIS2_PLACEMENT_3D('',#106312,#60315,#60316);
#49921=AXIS2_PLACEMENT_3D('',#106313,#60317,#60318);
#49922=AXIS2_PLACEMENT_3D('',#106318,#60320,#60321);
#49923=AXIS2_PLACEMENT_3D('',#106321,#60323,#60324);
#49924=AXIS2_PLACEMENT_3D('',#106322,#60325,#60326);
#49925=AXIS2_PLACEMENT_3D('',#106327,#60328,#60329);
#49926=AXIS2_PLACEMENT_3D('',#106330,#60331,#60332);
#49927=AXIS2_PLACEMENT_3D('',#106331,#60333,#60334);
#49928=AXIS2_PLACEMENT_3D('',#106336,#60336,#60337);
#49929=AXIS2_PLACEMENT_3D('',#106339,#60339,#60340);
#49930=AXIS2_PLACEMENT_3D('',#106340,#60341,#60342);
#49931=AXIS2_PLACEMENT_3D('',#106345,#60344,#60345);
#49932=AXIS2_PLACEMENT_3D('',#106348,#60347,#60348);
#49933=AXIS2_PLACEMENT_3D('',#106349,#60349,#60350);
#49934=AXIS2_PLACEMENT_3D('',#106354,#60352,#60353);
#49935=AXIS2_PLACEMENT_3D('',#106357,#60355,#60356);
#49936=AXIS2_PLACEMENT_3D('',#106358,#60357,#60358);
#49937=AXIS2_PLACEMENT_3D('',#106363,#60360,#60361);
#49938=AXIS2_PLACEMENT_3D('',#106366,#60363,#60364);
#49939=AXIS2_PLACEMENT_3D('',#106367,#60365,#60366);
#49940=AXIS2_PLACEMENT_3D('',#106372,#60368,#60369);
#49941=AXIS2_PLACEMENT_3D('',#106375,#60371,#60372);
#49942=AXIS2_PLACEMENT_3D('',#106376,#60373,#60374);
#49943=AXIS2_PLACEMENT_3D('',#106381,#60376,#60377);
#49944=AXIS2_PLACEMENT_3D('',#106384,#60379,#60380);
#49945=AXIS2_PLACEMENT_3D('',#106385,#60381,#60382);
#49946=AXIS2_PLACEMENT_3D('',#106390,#60384,#60385);
#49947=AXIS2_PLACEMENT_3D('',#106393,#60387,#60388);
#49948=AXIS2_PLACEMENT_3D('',#106394,#60389,#60390);
#49949=AXIS2_PLACEMENT_3D('',#106399,#60392,#60393);
#49950=AXIS2_PLACEMENT_3D('',#106402,#60395,#60396);
#49951=AXIS2_PLACEMENT_3D('',#106403,#60397,#60398);
#49952=AXIS2_PLACEMENT_3D('',#106408,#60400,#60401);
#49953=AXIS2_PLACEMENT_3D('',#106411,#60403,#60404);
#49954=AXIS2_PLACEMENT_3D('',#106412,#60405,#60406);
#49955=AXIS2_PLACEMENT_3D('',#106417,#60408,#60409);
#49956=AXIS2_PLACEMENT_3D('',#106420,#60411,#60412);
#49957=AXIS2_PLACEMENT_3D('',#106421,#60413,#60414);
#49958=AXIS2_PLACEMENT_3D('',#106426,#60416,#60417);
#49959=AXIS2_PLACEMENT_3D('',#106429,#60419,#60420);
#49960=AXIS2_PLACEMENT_3D('',#106430,#60421,#60422);
#49961=AXIS2_PLACEMENT_3D('',#106435,#60424,#60425);
#49962=AXIS2_PLACEMENT_3D('',#106438,#60427,#60428);
#49963=AXIS2_PLACEMENT_3D('',#106439,#60429,#60430);
#49964=AXIS2_PLACEMENT_3D('',#106444,#60432,#60433);
#49965=AXIS2_PLACEMENT_3D('',#106447,#60435,#60436);
#49966=AXIS2_PLACEMENT_3D('',#106448,#60437,#60438);
#49967=AXIS2_PLACEMENT_3D('',#106453,#60440,#60441);
#49968=AXIS2_PLACEMENT_3D('',#106456,#60443,#60444);
#49969=AXIS2_PLACEMENT_3D('',#106457,#60445,#60446);
#49970=AXIS2_PLACEMENT_3D('',#106462,#60448,#60449);
#49971=AXIS2_PLACEMENT_3D('',#106465,#60451,#60452);
#49972=AXIS2_PLACEMENT_3D('',#106466,#60453,#60454);
#49973=AXIS2_PLACEMENT_3D('',#106471,#60456,#60457);
#49974=AXIS2_PLACEMENT_3D('',#106474,#60459,#60460);
#49975=AXIS2_PLACEMENT_3D('',#106475,#60461,#60462);
#49976=AXIS2_PLACEMENT_3D('',#106480,#60464,#60465);
#49977=AXIS2_PLACEMENT_3D('',#106483,#60467,#60468);
#49978=AXIS2_PLACEMENT_3D('',#106484,#60469,#60470);
#49979=AXIS2_PLACEMENT_3D('',#106489,#60472,#60473);
#49980=AXIS2_PLACEMENT_3D('',#106492,#60475,#60476);
#49981=AXIS2_PLACEMENT_3D('',#106493,#60477,#60478);
#49982=AXIS2_PLACEMENT_3D('',#106498,#60480,#60481);
#49983=AXIS2_PLACEMENT_3D('',#106501,#60483,#60484);
#49984=AXIS2_PLACEMENT_3D('',#106502,#60485,#60486);
#49985=AXIS2_PLACEMENT_3D('',#106507,#60488,#60489);
#49986=AXIS2_PLACEMENT_3D('',#106510,#60491,#60492);
#49987=AXIS2_PLACEMENT_3D('',#106511,#60493,#60494);
#49988=AXIS2_PLACEMENT_3D('',#106516,#60496,#60497);
#49989=AXIS2_PLACEMENT_3D('',#106519,#60499,#60500);
#49990=AXIS2_PLACEMENT_3D('',#106520,#60501,#60502);
#49991=AXIS2_PLACEMENT_3D('',#106525,#60504,#60505);
#49992=AXIS2_PLACEMENT_3D('',#106528,#60507,#60508);
#49993=AXIS2_PLACEMENT_3D('',#106529,#60509,#60510);
#49994=AXIS2_PLACEMENT_3D('',#106534,#60512,#60513);
#49995=AXIS2_PLACEMENT_3D('',#106537,#60515,#60516);
#49996=AXIS2_PLACEMENT_3D('',#106538,#60517,#60518);
#49997=AXIS2_PLACEMENT_3D('',#106543,#60520,#60521);
#49998=AXIS2_PLACEMENT_3D('',#106546,#60523,#60524);
#49999=AXIS2_PLACEMENT_3D('',#106547,#60525,#60526);
#50000=AXIS2_PLACEMENT_3D('',#106552,#60528,#60529);
#50001=AXIS2_PLACEMENT_3D('',#106555,#60531,#60532);
#50002=AXIS2_PLACEMENT_3D('',#106556,#60533,#60534);
#50003=AXIS2_PLACEMENT_3D('',#106561,#60536,#60537);
#50004=AXIS2_PLACEMENT_3D('',#106564,#60539,#60540);
#50005=AXIS2_PLACEMENT_3D('',#106565,#60541,#60542);
#50006=AXIS2_PLACEMENT_3D('',#106570,#60544,#60545);
#50007=AXIS2_PLACEMENT_3D('',#106573,#60547,#60548);
#50008=AXIS2_PLACEMENT_3D('',#106574,#60549,#60550);
#50009=AXIS2_PLACEMENT_3D('',#106579,#60552,#60553);
#50010=AXIS2_PLACEMENT_3D('',#106582,#60555,#60556);
#50011=AXIS2_PLACEMENT_3D('',#106583,#60557,#60558);
#50012=AXIS2_PLACEMENT_3D('',#106588,#60560,#60561);
#50013=AXIS2_PLACEMENT_3D('',#106591,#60563,#60564);
#50014=AXIS2_PLACEMENT_3D('',#106592,#60565,#60566);
#50015=AXIS2_PLACEMENT_3D('',#106597,#60568,#60569);
#50016=AXIS2_PLACEMENT_3D('',#106600,#60571,#60572);
#50017=AXIS2_PLACEMENT_3D('',#106601,#60573,#60574);
#50018=AXIS2_PLACEMENT_3D('',#106606,#60576,#60577);
#50019=AXIS2_PLACEMENT_3D('',#106609,#60579,#60580);
#50020=AXIS2_PLACEMENT_3D('',#106610,#60581,#60582);
#50021=AXIS2_PLACEMENT_3D('',#106615,#60584,#60585);
#50022=AXIS2_PLACEMENT_3D('',#106618,#60587,#60588);
#50023=AXIS2_PLACEMENT_3D('',#106619,#60589,#60590);
#50024=AXIS2_PLACEMENT_3D('',#106624,#60592,#60593);
#50025=AXIS2_PLACEMENT_3D('',#106627,#60595,#60596);
#50026=AXIS2_PLACEMENT_3D('',#106628,#60597,#60598);
#50027=AXIS2_PLACEMENT_3D('',#106633,#60600,#60601);
#50028=AXIS2_PLACEMENT_3D('',#106636,#60603,#60604);
#50029=AXIS2_PLACEMENT_3D('',#106637,#60605,#60606);
#50030=AXIS2_PLACEMENT_3D('',#106642,#60608,#60609);
#50031=AXIS2_PLACEMENT_3D('',#106645,#60611,#60612);
#50032=AXIS2_PLACEMENT_3D('',#106646,#60613,#60614);
#50033=AXIS2_PLACEMENT_3D('',#106651,#60616,#60617);
#50034=AXIS2_PLACEMENT_3D('',#106654,#60619,#60620);
#50035=AXIS2_PLACEMENT_3D('',#106655,#60621,#60622);
#50036=AXIS2_PLACEMENT_3D('',#106660,#60624,#60625);
#50037=AXIS2_PLACEMENT_3D('',#106663,#60627,#60628);
#50038=AXIS2_PLACEMENT_3D('',#106664,#60629,#60630);
#50039=AXIS2_PLACEMENT_3D('',#106669,#60632,#60633);
#50040=AXIS2_PLACEMENT_3D('',#106672,#60635,#60636);
#50041=AXIS2_PLACEMENT_3D('',#106673,#60637,#60638);
#50042=AXIS2_PLACEMENT_3D('',#106678,#60640,#60641);
#50043=AXIS2_PLACEMENT_3D('',#106681,#60643,#60644);
#50044=AXIS2_PLACEMENT_3D('',#106682,#60645,#60646);
#50045=AXIS2_PLACEMENT_3D('',#106687,#60648,#60649);
#50046=AXIS2_PLACEMENT_3D('',#106690,#60651,#60652);
#50047=AXIS2_PLACEMENT_3D('',#106691,#60653,#60654);
#50048=AXIS2_PLACEMENT_3D('',#106696,#60656,#60657);
#50049=AXIS2_PLACEMENT_3D('',#106699,#60659,#60660);
#50050=AXIS2_PLACEMENT_3D('',#106700,#60661,#60662);
#50051=AXIS2_PLACEMENT_3D('',#106705,#60664,#60665);
#50052=AXIS2_PLACEMENT_3D('',#106708,#60667,#60668);
#50053=AXIS2_PLACEMENT_3D('',#106709,#60669,#60670);
#50054=AXIS2_PLACEMENT_3D('',#106714,#60672,#60673);
#50055=AXIS2_PLACEMENT_3D('',#106717,#60675,#60676);
#50056=AXIS2_PLACEMENT_3D('',#106718,#60677,#60678);
#50057=AXIS2_PLACEMENT_3D('',#106723,#60680,#60681);
#50058=AXIS2_PLACEMENT_3D('',#106726,#60683,#60684);
#50059=AXIS2_PLACEMENT_3D('',#106727,#60685,#60686);
#50060=AXIS2_PLACEMENT_3D('',#106732,#60688,#60689);
#50061=AXIS2_PLACEMENT_3D('',#106735,#60691,#60692);
#50062=AXIS2_PLACEMENT_3D('',#106736,#60693,#60694);
#50063=AXIS2_PLACEMENT_3D('',#106741,#60696,#60697);
#50064=AXIS2_PLACEMENT_3D('',#106744,#60699,#60700);
#50065=AXIS2_PLACEMENT_3D('',#106745,#60701,#60702);
#50066=AXIS2_PLACEMENT_3D('',#106899,#60805,#60806);
#50067=AXIS2_PLACEMENT_3D('',#107053,#60909,#60910);
#50068=AXIS2_PLACEMENT_3D('',#107054,#60911,#60912);
#50069=AXIS2_PLACEMENT_3D('',#107055,#60913,#60914);
#50070=AXIS2_PLACEMENT_3D('',#107056,#60915,#60916);
#50071=AXIS2_PLACEMENT_3D('',#107057,#60917,#60918);
#50072=AXIS2_PLACEMENT_3D('',#107059,#60920,#60921);
#50073=AXIS2_PLACEMENT_3D('',#107060,#60922,#60923);
#50074=AXIS2_PLACEMENT_3D('',#107062,#60925,#60926);
#50075=AXIS2_PLACEMENT_3D('',#107063,#60927,#60928);
#50076=AXIS2_PLACEMENT_3D('',#107065,#60930,#60931);
#50077=AXIS2_PLACEMENT_3D('',#107066,#60932,#60933);
#50078=AXIS2_PLACEMENT_3D('',#107068,#60935,#60936);
#50079=AXIS2_PLACEMENT_3D('',#107069,#60937,#60938);
#50080=AXIS2_PLACEMENT_3D('',#107071,#60940,#60941);
#50081=AXIS2_PLACEMENT_3D('',#107072,#60942,#60943);
#50082=AXIS2_PLACEMENT_3D('',#107074,#60945,#60946);
#50083=AXIS2_PLACEMENT_3D('',#107075,#60947,#60948);
#50084=AXIS2_PLACEMENT_3D('',#107077,#60950,#60951);
#50085=AXIS2_PLACEMENT_3D('',#107078,#60952,#60953);
#50086=AXIS2_PLACEMENT_3D('',#107080,#60955,#60956);
#50087=AXIS2_PLACEMENT_3D('',#107081,#60957,#60958);
#50088=AXIS2_PLACEMENT_3D('',#107083,#60960,#60961);
#50089=AXIS2_PLACEMENT_3D('',#107084,#60962,#60963);
#50090=AXIS2_PLACEMENT_3D('',#107086,#60965,#60966);
#50091=AXIS2_PLACEMENT_3D('',#107087,#60967,#60968);
#50092=AXIS2_PLACEMENT_3D('',#107089,#60970,#60971);
#50093=AXIS2_PLACEMENT_3D('',#107090,#60972,#60973);
#50094=AXIS2_PLACEMENT_3D('',#107092,#60975,#60976);
#50095=AXIS2_PLACEMENT_3D('',#107093,#60977,#60978);
#50096=AXIS2_PLACEMENT_3D('',#107095,#60980,#60981);
#50097=AXIS2_PLACEMENT_3D('',#107096,#60982,#60983);
#50098=AXIS2_PLACEMENT_3D('',#107098,#60985,#60986);
#50099=AXIS2_PLACEMENT_3D('',#107099,#60987,#60988);
#50100=AXIS2_PLACEMENT_3D('',#107101,#60990,#60991);
#50101=AXIS2_PLACEMENT_3D('',#107102,#60992,#60993);
#50102=AXIS2_PLACEMENT_3D('',#107104,#60995,#60996);
#50103=AXIS2_PLACEMENT_3D('',#107105,#60997,#60998);
#50104=AXIS2_PLACEMENT_3D('',#107107,#61000,#61001);
#50105=AXIS2_PLACEMENT_3D('',#107108,#61002,#61003);
#50106=AXIS2_PLACEMENT_3D('',#107110,#61005,#61006);
#50107=AXIS2_PLACEMENT_3D('',#107111,#61007,#61008);
#50108=AXIS2_PLACEMENT_3D('',#107113,#61010,#61011);
#50109=AXIS2_PLACEMENT_3D('',#107114,#61012,#61013);
#50110=AXIS2_PLACEMENT_3D('',#107116,#61015,#61016);
#50111=AXIS2_PLACEMENT_3D('',#107117,#61017,#61018);
#50112=AXIS2_PLACEMENT_3D('',#107119,#61020,#61021);
#50113=AXIS2_PLACEMENT_3D('',#107120,#61022,#61023);
#50114=AXIS2_PLACEMENT_3D('',#107122,#61025,#61026);
#50115=AXIS2_PLACEMENT_3D('',#107123,#61027,#61028);
#50116=AXIS2_PLACEMENT_3D('',#107125,#61030,#61031);
#50117=AXIS2_PLACEMENT_3D('',#107126,#61032,#61033);
#50118=AXIS2_PLACEMENT_3D('',#107128,#61035,#61036);
#50119=AXIS2_PLACEMENT_3D('',#107129,#61037,#61038);
#50120=AXIS2_PLACEMENT_3D('',#107131,#61040,#61041);
#50121=AXIS2_PLACEMENT_3D('',#107132,#61042,#61043);
#50122=AXIS2_PLACEMENT_3D('',#107134,#61045,#61046);
#50123=AXIS2_PLACEMENT_3D('',#107135,#61047,#61048);
#50124=AXIS2_PLACEMENT_3D('',#107137,#61050,#61051);
#50125=AXIS2_PLACEMENT_3D('',#107138,#61052,#61053);
#50126=AXIS2_PLACEMENT_3D('',#107140,#61055,#61056);
#50127=AXIS2_PLACEMENT_3D('',#107141,#61057,#61058);
#50128=AXIS2_PLACEMENT_3D('',#107143,#61060,#61061);
#50129=AXIS2_PLACEMENT_3D('',#107144,#61062,#61063);
#50130=AXIS2_PLACEMENT_3D('',#107146,#61065,#61066);
#50131=AXIS2_PLACEMENT_3D('',#107147,#61067,#61068);
#50132=AXIS2_PLACEMENT_3D('',#107149,#61070,#61071);
#50133=AXIS2_PLACEMENT_3D('',#107150,#61072,#61073);
#50134=AXIS2_PLACEMENT_3D('',#107152,#61075,#61076);
#50135=AXIS2_PLACEMENT_3D('',#107153,#61077,#61078);
#50136=AXIS2_PLACEMENT_3D('',#107155,#61080,#61081);
#50137=AXIS2_PLACEMENT_3D('',#107156,#61082,#61083);
#50138=AXIS2_PLACEMENT_3D('',#107158,#61085,#61086);
#50139=AXIS2_PLACEMENT_3D('',#107159,#61087,#61088);
#50140=AXIS2_PLACEMENT_3D('',#107161,#61090,#61091);
#50141=AXIS2_PLACEMENT_3D('',#107162,#61092,#61093);
#50142=AXIS2_PLACEMENT_3D('',#107164,#61095,#61096);
#50143=AXIS2_PLACEMENT_3D('',#107165,#61097,#61098);
#50144=AXIS2_PLACEMENT_3D('',#107167,#61100,#61101);
#50145=AXIS2_PLACEMENT_3D('',#107168,#61102,#61103);
#50146=AXIS2_PLACEMENT_3D('',#107170,#61105,#61106);
#50147=AXIS2_PLACEMENT_3D('',#107171,#61107,#61108);
#50148=AXIS2_PLACEMENT_3D('',#107173,#61110,#61111);
#50149=AXIS2_PLACEMENT_3D('',#107174,#61112,#61113);
#50150=AXIS2_PLACEMENT_3D('',#107176,#61115,#61116);
#50151=AXIS2_PLACEMENT_3D('',#107177,#61117,#61118);
#50152=AXIS2_PLACEMENT_3D('',#107179,#61120,#61121);
#50153=AXIS2_PLACEMENT_3D('',#107180,#61122,#61123);
#50154=AXIS2_PLACEMENT_3D('',#107182,#61125,#61126);
#50155=AXIS2_PLACEMENT_3D('',#107183,#61127,#61128);
#50156=AXIS2_PLACEMENT_3D('',#107185,#61130,#61131);
#50157=AXIS2_PLACEMENT_3D('',#107186,#61132,#61133);
#50158=AXIS2_PLACEMENT_3D('',#107188,#61135,#61136);
#50159=AXIS2_PLACEMENT_3D('',#107189,#61137,#61138);
#50160=AXIS2_PLACEMENT_3D('',#107191,#61140,#61141);
#50161=AXIS2_PLACEMENT_3D('',#107192,#61142,#61143);
#50162=AXIS2_PLACEMENT_3D('',#107194,#61145,#61146);
#50163=AXIS2_PLACEMENT_3D('',#107195,#61147,#61148);
#50164=AXIS2_PLACEMENT_3D('',#107197,#61150,#61151);
#50165=AXIS2_PLACEMENT_3D('',#107198,#61152,#61153);
#50166=AXIS2_PLACEMENT_3D('',#107200,#61155,#61156);
#50167=AXIS2_PLACEMENT_3D('',#107201,#61157,#61158);
#50168=AXIS2_PLACEMENT_3D('',#107203,#61160,#61161);
#50169=AXIS2_PLACEMENT_3D('',#107204,#61162,#61163);
#50170=AXIS2_PLACEMENT_3D('',#107206,#61165,#61166);
#50171=AXIS2_PLACEMENT_3D('',#107207,#61167,#61168);
#50172=AXIS2_PLACEMENT_3D('',#107209,#61170,#61171);
#60263=DIRECTION('axis',(0.,0.,1.));
#60264=DIRECTION('refdir',(1.,0.,0.));
#60265=DIRECTION('center_axis',(0.,0.,1.));
#60266=DIRECTION('ref_axis',(1.,0.,0.));
#60267=DIRECTION('center_axis',(0.,0.,-1.));
#60268=DIRECTION('ref_axis',(-1.,0.,0.));
#60269=DIRECTION('',(0.,0.,-1.));
#60270=DIRECTION('center_axis',(0.,0.,-1.));
#60271=DIRECTION('ref_axis',(-1.,0.,0.));
#60272=DIRECTION('center_axis',(0.,0.,-1.));
#60273=DIRECTION('ref_axis',(-1.,0.,0.));
#60274=DIRECTION('center_axis',(0.,0.,1.));
#60275=DIRECTION('ref_axis',(1.,0.,0.));
#60276=DIRECTION('',(0.,0.,1.));
#60277=DIRECTION('center_axis',(0.,0.,1.));
#60278=DIRECTION('ref_axis',(1.,0.,0.));
#60279=DIRECTION('center_axis',(0.,0.,1.));
#60280=DIRECTION('ref_axis',(1.,0.,0.));
#60281=DIRECTION('center_axis',(0.,0.,1.));
#60282=DIRECTION('ref_axis',(1.,0.,0.));
#60283=DIRECTION('',(0.,0.,1.));
#60284=DIRECTION('center_axis',(0.,0.,1.));
#60285=DIRECTION('ref_axis',(1.,0.,0.));
#60286=DIRECTION('center_axis',(0.,0.,-1.));
#60287=DIRECTION('ref_axis',(-1.,0.,0.));
#60288=DIRECTION('center_axis',(0.,0.,-1.));
#60289=DIRECTION('ref_axis',(-1.,0.,0.));
#60290=DIRECTION('',(0.,0.,-1.));
#60291=DIRECTION('center_axis',(0.,0.,-1.));
#60292=DIRECTION('ref_axis',(-1.,0.,0.));
#60293=DIRECTION('center_axis',(0.,0.,-1.));
#60294=DIRECTION('ref_axis',(-1.,0.,0.));
#60295=DIRECTION('',(0.,0.,-1.));
#60296=DIRECTION('center_axis',(0.,0.,-1.));
#60297=DIRECTION('ref_axis',(-1.,0.,0.));
#60298=DIRECTION('',(0.,0.,-1.));
#60299=DIRECTION('center_axis',(0.,0.,-1.));
#60300=DIRECTION('ref_axis',(-1.,0.,0.));
#60301=DIRECTION('center_axis',(0.,0.,-1.));
#60302=DIRECTION('ref_axis',(-1.,0.,0.));
#60303=DIRECTION('',(0.,0.,-1.));
#60304=DIRECTION('center_axis',(0.,0.,-1.));
#60305=DIRECTION('ref_axis',(-1.,0.,0.));
#60306=DIRECTION('',(0.,0.,-1.));
#60307=DIRECTION('center_axis',(0.,0.,-1.));
#60308=DIRECTION('ref_axis',(-1.,0.,0.));
#60309=DIRECTION('center_axis',(0.,0.,-1.));
#60310=DIRECTION('ref_axis',(-1.,0.,0.));
#60311=DIRECTION('',(0.,0.,-1.));
#60312=DIRECTION('center_axis',(0.,0.,-1.));
#60313=DIRECTION('ref_axis',(-1.,0.,0.));
#60314=DIRECTION('',(0.,0.,-1.));
#60315=DIRECTION('center_axis',(0.,0.,-1.));
#60316=DIRECTION('ref_axis',(-1.,0.,0.));
#60317=DIRECTION('center_axis',(0.,0.,-1.));
#60318=DIRECTION('ref_axis',(-1.,0.,0.));
#60319=DIRECTION('',(0.,0.,-1.));
#60320=DIRECTION('center_axis',(0.,0.,-1.));
#60321=DIRECTION('ref_axis',(-1.,0.,0.));
#60322=DIRECTION('',(0.,0.,-1.));
#60323=DIRECTION('center_axis',(0.,0.,-1.));
#60324=DIRECTION('ref_axis',(-1.,0.,0.));
#60325=DIRECTION('center_axis',(0.,0.,-1.));
#60326=DIRECTION('ref_axis',(-1.,0.,0.));
#60327=DIRECTION('',(0.,0.,-1.));
#60328=DIRECTION('center_axis',(0.,0.,-1.));
#60329=DIRECTION('ref_axis',(-1.,0.,0.));
#60330=DIRECTION('',(0.,0.,-1.));
#60331=DIRECTION('center_axis',(0.,0.,-1.));
#60332=DIRECTION('ref_axis',(-1.,0.,0.));
#60333=DIRECTION('center_axis',(0.,0.,-1.));
#60334=DIRECTION('ref_axis',(-1.,0.,0.));
#60335=DIRECTION('',(0.,0.,-1.));
#60336=DIRECTION('center_axis',(0.,0.,-1.));
#60337=DIRECTION('ref_axis',(-1.,0.,0.));
#60338=DIRECTION('',(0.,0.,-1.));
#60339=DIRECTION('center_axis',(0.,0.,-1.));
#60340=DIRECTION('ref_axis',(-1.,0.,0.));
#60341=DIRECTION('center_axis',(0.,0.,-1.));
#60342=DIRECTION('ref_axis',(-1.,0.,0.));
#60343=DIRECTION('',(0.,0.,-1.));
#60344=DIRECTION('center_axis',(0.,0.,-1.));
#60345=DIRECTION('ref_axis',(-1.,0.,0.));
#60346=DIRECTION('',(0.,0.,-1.));
#60347=DIRECTION('center_axis',(0.,0.,-1.));
#60348=DIRECTION('ref_axis',(-1.,0.,0.));
#60349=DIRECTION('center_axis',(0.,0.,-1.));
#60350=DIRECTION('ref_axis',(-1.,0.,0.));
#60351=DIRECTION('',(0.,0.,-1.));
#60352=DIRECTION('center_axis',(0.,0.,-1.));
#60353=DIRECTION('ref_axis',(-1.,0.,0.));
#60354=DIRECTION('',(0.,0.,-1.));
#60355=DIRECTION('center_axis',(0.,0.,-1.));
#60356=DIRECTION('ref_axis',(-1.,0.,0.));
#60357=DIRECTION('center_axis',(0.,0.,-1.));
#60358=DIRECTION('ref_axis',(-1.,0.,0.));
#60359=DIRECTION('',(0.,0.,-1.));
#60360=DIRECTION('center_axis',(0.,0.,-1.));
#60361=DIRECTION('ref_axis',(-1.,0.,0.));
#60362=DIRECTION('',(0.,0.,-1.));
#60363=DIRECTION('center_axis',(0.,0.,-1.));
#60364=DIRECTION('ref_axis',(-1.,0.,0.));
#60365=DIRECTION('center_axis',(0.,0.,-1.));
#60366=DIRECTION('ref_axis',(-1.,0.,0.));
#60367=DIRECTION('',(0.,0.,-1.));
#60368=DIRECTION('center_axis',(0.,0.,-1.));
#60369=DIRECTION('ref_axis',(-1.,0.,0.));
#60370=DIRECTION('',(0.,0.,-1.));
#60371=DIRECTION('center_axis',(0.,0.,-1.));
#60372=DIRECTION('ref_axis',(-1.,0.,0.));
#60373=DIRECTION('center_axis',(0.,0.,-1.));
#60374=DIRECTION('ref_axis',(-1.,0.,0.));
#60375=DIRECTION('',(0.,0.,-1.));
#60376=DIRECTION('center_axis',(0.,0.,-1.));
#60377=DIRECTION('ref_axis',(-1.,0.,0.));
#60378=DIRECTION('',(0.,0.,-1.));
#60379=DIRECTION('center_axis',(0.,0.,-1.));
#60380=DIRECTION('ref_axis',(-1.,0.,0.));
#60381=DIRECTION('center_axis',(0.,0.,-1.));
#60382=DIRECTION('ref_axis',(-1.,0.,0.));
#60383=DIRECTION('',(0.,0.,-1.));
#60384=DIRECTION('center_axis',(0.,0.,-1.));
#60385=DIRECTION('ref_axis',(-1.,0.,0.));
#60386=DIRECTION('',(0.,0.,-1.));
#60387=DIRECTION('center_axis',(0.,0.,-1.));
#60388=DIRECTION('ref_axis',(-1.,0.,0.));
#60389=DIRECTION('center_axis',(0.,0.,-1.));
#60390=DIRECTION('ref_axis',(-1.,0.,0.));
#60391=DIRECTION('',(0.,0.,-1.));
#60392=DIRECTION('center_axis',(0.,0.,-1.));
#60393=DIRECTION('ref_axis',(-1.,0.,0.));
#60394=DIRECTION('',(0.,0.,-1.));
#60395=DIRECTION('center_axis',(0.,0.,-1.));
#60396=DIRECTION('ref_axis',(-1.,0.,0.));
#60397=DIRECTION('center_axis',(0.,0.,-1.));
#60398=DIRECTION('ref_axis',(-1.,0.,0.));
#60399=DIRECTION('',(0.,0.,-1.));
#60400=DIRECTION('center_axis',(0.,0.,-1.));
#60401=DIRECTION('ref_axis',(-1.,0.,0.));
#60402=DIRECTION('',(0.,0.,-1.));
#60403=DIRECTION('center_axis',(0.,0.,-1.));
#60404=DIRECTION('ref_axis',(-1.,0.,0.));
#60405=DIRECTION('center_axis',(0.,0.,-1.));
#60406=DIRECTION('ref_axis',(-1.,0.,0.));
#60407=DIRECTION('',(0.,0.,-1.));
#60408=DIRECTION('center_axis',(0.,0.,-1.));
#60409=DIRECTION('ref_axis',(-1.,0.,0.));
#60410=DIRECTION('',(0.,0.,-1.));
#60411=DIRECTION('center_axis',(0.,0.,-1.));
#60412=DIRECTION('ref_axis',(-1.,0.,0.));
#60413=DIRECTION('center_axis',(0.,0.,-1.));
#60414=DIRECTION('ref_axis',(-1.,0.,0.));
#60415=DIRECTION('',(0.,0.,-1.));
#60416=DIRECTION('center_axis',(0.,0.,-1.));
#60417=DIRECTION('ref_axis',(-1.,0.,0.));
#60418=DIRECTION('',(0.,0.,-1.));
#60419=DIRECTION('center_axis',(0.,0.,-1.));
#60420=DIRECTION('ref_axis',(-1.,0.,0.));
#60421=DIRECTION('center_axis',(0.,0.,-1.));
#60422=DIRECTION('ref_axis',(-1.,0.,0.));
#60423=DIRECTION('',(0.,0.,-1.));
#60424=DIRECTION('center_axis',(0.,0.,-1.));
#60425=DIRECTION('ref_axis',(-1.,0.,0.));
#60426=DIRECTION('',(0.,0.,-1.));
#60427=DIRECTION('center_axis',(0.,0.,-1.));
#60428=DIRECTION('ref_axis',(-1.,0.,0.));
#60429=DIRECTION('center_axis',(0.,0.,-1.));
#60430=DIRECTION('ref_axis',(-1.,0.,0.));
#60431=DIRECTION('',(0.,0.,-1.));
#60432=DIRECTION('center_axis',(0.,0.,-1.));
#60433=DIRECTION('ref_axis',(-1.,0.,0.));
#60434=DIRECTION('',(0.,0.,-1.));
#60435=DIRECTION('center_axis',(0.,0.,-1.));
#60436=DIRECTION('ref_axis',(-1.,0.,0.));
#60437=DIRECTION('center_axis',(0.,0.,-1.));
#60438=DIRECTION('ref_axis',(-1.,0.,0.));
#60439=DIRECTION('',(0.,0.,-1.));
#60440=DIRECTION('center_axis',(0.,0.,-1.));
#60441=DIRECTION('ref_axis',(-1.,0.,0.));
#60442=DIRECTION('',(0.,0.,-1.));
#60443=DIRECTION('center_axis',(0.,0.,-1.));
#60444=DIRECTION('ref_axis',(-1.,0.,0.));
#60445=DIRECTION('center_axis',(0.,0.,-1.));
#60446=DIRECTION('ref_axis',(-1.,0.,0.));
#60447=DIRECTION('',(0.,0.,-1.));
#60448=DIRECTION('center_axis',(0.,0.,-1.));
#60449=DIRECTION('ref_axis',(-1.,0.,0.));
#60450=DIRECTION('',(0.,0.,-1.));
#60451=DIRECTION('center_axis',(0.,0.,-1.));
#60452=DIRECTION('ref_axis',(-1.,0.,0.));
#60453=DIRECTION('center_axis',(0.,0.,-1.));
#60454=DIRECTION('ref_axis',(-1.,0.,0.));
#60455=DIRECTION('',(0.,0.,-1.));
#60456=DIRECTION('center_axis',(0.,0.,-1.));
#60457=DIRECTION('ref_axis',(-1.,0.,0.));
#60458=DIRECTION('',(0.,0.,-1.));
#60459=DIRECTION('center_axis',(0.,0.,-1.));
#60460=DIRECTION('ref_axis',(-1.,0.,0.));
#60461=DIRECTION('center_axis',(0.,0.,-1.));
#60462=DIRECTION('ref_axis',(-1.,0.,0.));
#60463=DIRECTION('',(0.,0.,-1.));
#60464=DIRECTION('center_axis',(0.,0.,-1.));
#60465=DIRECTION('ref_axis',(-1.,0.,0.));
#60466=DIRECTION('',(0.,0.,-1.));
#60467=DIRECTION('center_axis',(0.,0.,-1.));
#60468=DIRECTION('ref_axis',(-1.,0.,0.));
#60469=DIRECTION('center_axis',(0.,0.,-1.));
#60470=DIRECTION('ref_axis',(-1.,0.,0.));
#60471=DIRECTION('',(0.,0.,-1.));
#60472=DIRECTION('center_axis',(0.,0.,-1.));
#60473=DIRECTION('ref_axis',(-1.,0.,0.));
#60474=DIRECTION('',(0.,0.,-1.));
#60475=DIRECTION('center_axis',(0.,0.,-1.));
#60476=DIRECTION('ref_axis',(-1.,0.,0.));
#60477=DIRECTION('center_axis',(0.,0.,-1.));
#60478=DIRECTION('ref_axis',(-1.,0.,0.));
#60479=DIRECTION('',(0.,0.,-1.));
#60480=DIRECTION('center_axis',(0.,0.,-1.));
#60481=DIRECTION('ref_axis',(-1.,0.,0.));
#60482=DIRECTION('',(0.,0.,-1.));
#60483=DIRECTION('center_axis',(0.,0.,-1.));
#60484=DIRECTION('ref_axis',(-1.,0.,0.));
#60485=DIRECTION('center_axis',(0.,0.,-1.));
#60486=DIRECTION('ref_axis',(-1.,0.,0.));
#60487=DIRECTION('',(0.,0.,-1.));
#60488=DIRECTION('center_axis',(0.,0.,-1.));
#60489=DIRECTION('ref_axis',(-1.,0.,0.));
#60490=DIRECTION('',(0.,0.,-1.));
#60491=DIRECTION('center_axis',(0.,0.,-1.));
#60492=DIRECTION('ref_axis',(-1.,0.,0.));
#60493=DIRECTION('center_axis',(0.,0.,-1.));
#60494=DIRECTION('ref_axis',(-1.,0.,0.));
#60495=DIRECTION('',(0.,0.,-1.));
#60496=DIRECTION('center_axis',(0.,0.,-1.));
#60497=DIRECTION('ref_axis',(-1.,0.,0.));
#60498=DIRECTION('',(0.,0.,-1.));
#60499=DIRECTION('center_axis',(0.,0.,-1.));
#60500=DIRECTION('ref_axis',(-1.,0.,0.));
#60501=DIRECTION('center_axis',(0.,0.,-1.));
#60502=DIRECTION('ref_axis',(-1.,0.,0.));
#60503=DIRECTION('',(0.,0.,-1.));
#60504=DIRECTION('center_axis',(0.,0.,-1.));
#60505=DIRECTION('ref_axis',(-1.,0.,0.));
#60506=DIRECTION('',(0.,0.,-1.));
#60507=DIRECTION('center_axis',(0.,0.,-1.));
#60508=DIRECTION('ref_axis',(-1.,0.,0.));
#60509=DIRECTION('center_axis',(0.,0.,-1.));
#60510=DIRECTION('ref_axis',(-1.,0.,0.));
#60511=DIRECTION('',(0.,0.,-1.));
#60512=DIRECTION('center_axis',(0.,0.,-1.));
#60513=DIRECTION('ref_axis',(-1.,0.,0.));
#60514=DIRECTION('',(0.,0.,-1.));
#60515=DIRECTION('center_axis',(0.,0.,-1.));
#60516=DIRECTION('ref_axis',(-1.,0.,0.));
#60517=DIRECTION('center_axis',(0.,0.,-1.));
#60518=DIRECTION('ref_axis',(-1.,0.,0.));
#60519=DIRECTION('',(0.,0.,-1.));
#60520=DIRECTION('center_axis',(0.,0.,-1.));
#60521=DIRECTION('ref_axis',(-1.,0.,0.));
#60522=DIRECTION('',(0.,0.,-1.));
#60523=DIRECTION('center_axis',(0.,0.,-1.));
#60524=DIRECTION('ref_axis',(-1.,0.,0.));
#60525=DIRECTION('center_axis',(0.,0.,-1.));
#60526=DIRECTION('ref_axis',(-1.,0.,0.));
#60527=DIRECTION('',(0.,0.,-1.));
#60528=DIRECTION('center_axis',(0.,0.,-1.));
#60529=DIRECTION('ref_axis',(-1.,0.,0.));
#60530=DIRECTION('',(0.,0.,-1.));
#60531=DIRECTION('center_axis',(0.,0.,-1.));
#60532=DIRECTION('ref_axis',(-1.,0.,0.));
#60533=DIRECTION('center_axis',(0.,0.,-1.));
#60534=DIRECTION('ref_axis',(-1.,0.,0.));
#60535=DIRECTION('',(0.,0.,-1.));
#60536=DIRECTION('center_axis',(0.,0.,-1.));
#60537=DIRECTION('ref_axis',(-1.,0.,0.));
#60538=DIRECTION('',(0.,0.,-1.));
#60539=DIRECTION('center_axis',(0.,0.,-1.));
#60540=DIRECTION('ref_axis',(-1.,0.,0.));
#60541=DIRECTION('center_axis',(0.,0.,-1.));
#60542=DIRECTION('ref_axis',(-1.,0.,0.));
#60543=DIRECTION('',(0.,0.,-1.));
#60544=DIRECTION('center_axis',(0.,0.,-1.));
#60545=DIRECTION('ref_axis',(-1.,0.,0.));
#60546=DIRECTION('',(0.,0.,-1.));
#60547=DIRECTION('center_axis',(0.,0.,-1.));
#60548=DIRECTION('ref_axis',(-1.,0.,0.));
#60549=DIRECTION('center_axis',(0.,0.,-1.));
#60550=DIRECTION('ref_axis',(-1.,0.,0.));
#60551=DIRECTION('',(0.,0.,-1.));
#60552=DIRECTION('center_axis',(0.,0.,-1.));
#60553=DIRECTION('ref_axis',(-1.,0.,0.));
#60554=DIRECTION('',(0.,0.,-1.));
#60555=DIRECTION('center_axis',(0.,0.,-1.));
#60556=DIRECTION('ref_axis',(-1.,0.,0.));
#60557=DIRECTION('center_axis',(0.,0.,-1.));
#60558=DIRECTION('ref_axis',(-1.,0.,0.));
#60559=DIRECTION('',(0.,0.,-1.));
#60560=DIRECTION('center_axis',(0.,0.,-1.));
#60561=DIRECTION('ref_axis',(-1.,0.,0.));
#60562=DIRECTION('',(0.,0.,-1.));
#60563=DIRECTION('center_axis',(0.,0.,-1.));
#60564=DIRECTION('ref_axis',(-1.,0.,0.));
#60565=DIRECTION('center_axis',(0.,0.,-1.));
#60566=DIRECTION('ref_axis',(-1.,0.,0.));
#60567=DIRECTION('',(0.,0.,-1.));
#60568=DIRECTION('center_axis',(0.,0.,-1.));
#60569=DIRECTION('ref_axis',(-1.,0.,0.));
#60570=DIRECTION('',(0.,0.,-1.));
#60571=DIRECTION('center_axis',(0.,0.,-1.));
#60572=DIRECTION('ref_axis',(-1.,0.,0.));
#60573=DIRECTION('center_axis',(0.,0.,-1.));
#60574=DIRECTION('ref_axis',(-1.,0.,0.));
#60575=DIRECTION('',(0.,0.,-1.));
#60576=DIRECTION('center_axis',(0.,0.,-1.));
#60577=DIRECTION('ref_axis',(-1.,0.,0.));
#60578=DIRECTION('',(0.,0.,-1.));
#60579=DIRECTION('center_axis',(0.,0.,-1.));
#60580=DIRECTION('ref_axis',(-1.,0.,0.));
#60581=DIRECTION('center_axis',(0.,0.,-1.));
#60582=DIRECTION('ref_axis',(-1.,0.,0.));
#60583=DIRECTION('',(0.,0.,-1.));
#60584=DIRECTION('center_axis',(0.,0.,-1.));
#60585=DIRECTION('ref_axis',(-1.,0.,0.));
#60586=DIRECTION('',(0.,0.,-1.));
#60587=DIRECTION('center_axis',(0.,0.,-1.));
#60588=DIRECTION('ref_axis',(-1.,0.,0.));
#60589=DIRECTION('center_axis',(0.,0.,-1.));
#60590=DIRECTION('ref_axis',(-1.,0.,0.));
#60591=DIRECTION('',(0.,0.,-1.));
#60592=DIRECTION('center_axis',(0.,0.,-1.));
#60593=DIRECTION('ref_axis',(-1.,0.,0.));
#60594=DIRECTION('',(0.,0.,-1.));
#60595=DIRECTION('center_axis',(0.,0.,-1.));
#60596=DIRECTION('ref_axis',(-1.,0.,0.));
#60597=DIRECTION('center_axis',(0.,0.,-1.));
#60598=DIRECTION('ref_axis',(-1.,0.,0.));
#60599=DIRECTION('',(0.,0.,-1.));
#60600=DIRECTION('center_axis',(0.,0.,-1.));
#60601=DIRECTION('ref_axis',(-1.,0.,0.));
#60602=DIRECTION('',(0.,0.,-1.));
#60603=DIRECTION('center_axis',(0.,0.,-1.));
#60604=DIRECTION('ref_axis',(-1.,0.,0.));
#60605=DIRECTION('center_axis',(0.,0.,-1.));
#60606=DIRECTION('ref_axis',(-1.,0.,0.));
#60607=DIRECTION('',(0.,0.,-1.));
#60608=DIRECTION('center_axis',(0.,0.,-1.));
#60609=DIRECTION('ref_axis',(-1.,0.,0.));
#60610=DIRECTION('',(0.,0.,-1.));
#60611=DIRECTION('center_axis',(0.,0.,-1.));
#60612=DIRECTION('ref_axis',(-1.,0.,0.));
#60613=DIRECTION('center_axis',(0.,0.,-1.));
#60614=DIRECTION('ref_axis',(-1.,0.,0.));
#60615=DIRECTION('',(0.,0.,-1.));
#60616=DIRECTION('center_axis',(0.,0.,-1.));
#60617=DIRECTION('ref_axis',(-1.,0.,0.));
#60618=DIRECTION('',(0.,0.,-1.));
#60619=DIRECTION('center_axis',(0.,0.,-1.));
#60620=DIRECTION('ref_axis',(-1.,0.,0.));
#60621=DIRECTION('center_axis',(0.,0.,-1.));
#60622=DIRECTION('ref_axis',(-1.,0.,0.));
#60623=DIRECTION('',(0.,0.,-1.));
#60624=DIRECTION('center_axis',(0.,0.,-1.));
#60625=DIRECTION('ref_axis',(-1.,0.,0.));
#60626=DIRECTION('',(0.,0.,-1.));
#60627=DIRECTION('center_axis',(0.,0.,-1.));
#60628=DIRECTION('ref_axis',(-1.,0.,0.));
#60629=DIRECTION('center_axis',(0.,0.,-1.));
#60630=DIRECTION('ref_axis',(-1.,0.,0.));
#60631=DIRECTION('',(0.,0.,-1.));
#60632=DIRECTION('center_axis',(0.,0.,-1.));
#60633=DIRECTION('ref_axis',(-1.,0.,0.));
#60634=DIRECTION('',(0.,0.,-1.));
#60635=DIRECTION('center_axis',(0.,0.,-1.));
#60636=DIRECTION('ref_axis',(-1.,0.,0.));
#60637=DIRECTION('center_axis',(0.,0.,-1.));
#60638=DIRECTION('ref_axis',(-1.,0.,0.));
#60639=DIRECTION('',(0.,0.,-1.));
#60640=DIRECTION('center_axis',(0.,0.,-1.));
#60641=DIRECTION('ref_axis',(-1.,0.,0.));
#60642=DIRECTION('',(0.,0.,-1.));
#60643=DIRECTION('center_axis',(0.,0.,-1.));
#60644=DIRECTION('ref_axis',(-1.,0.,0.));
#60645=DIRECTION('center_axis',(0.,0.,-1.));
#60646=DIRECTION('ref_axis',(-1.,0.,0.));
#60647=DIRECTION('',(0.,0.,-1.));
#60648=DIRECTION('center_axis',(0.,0.,-1.));
#60649=DIRECTION('ref_axis',(-1.,0.,0.));
#60650=DIRECTION('',(0.,0.,-1.));
#60651=DIRECTION('center_axis',(0.,0.,-1.));
#60652=DIRECTION('ref_axis',(-1.,0.,0.));
#60653=DIRECTION('center_axis',(0.,0.,-1.));
#60654=DIRECTION('ref_axis',(-1.,0.,0.));
#60655=DIRECTION('',(0.,0.,-1.));
#60656=DIRECTION('center_axis',(0.,0.,-1.));
#60657=DIRECTION('ref_axis',(-1.,0.,0.));
#60658=DIRECTION('',(0.,0.,-1.));
#60659=DIRECTION('center_axis',(0.,0.,-1.));
#60660=DIRECTION('ref_axis',(-1.,0.,0.));
#60661=DIRECTION('center_axis',(0.,0.,-1.));
#60662=DIRECTION('ref_axis',(-1.,0.,0.));
#60663=DIRECTION('',(0.,0.,-1.));
#60664=DIRECTION('center_axis',(0.,0.,-1.));
#60665=DIRECTION('ref_axis',(-1.,0.,0.));
#60666=DIRECTION('',(0.,0.,-1.));
#60667=DIRECTION('center_axis',(0.,0.,-1.));
#60668=DIRECTION('ref_axis',(-1.,0.,0.));
#60669=DIRECTION('center_axis',(0.,0.,-1.));
#60670=DIRECTION('ref_axis',(-1.,0.,0.));
#60671=DIRECTION('',(0.,0.,-1.));
#60672=DIRECTION('center_axis',(0.,0.,-1.));
#60673=DIRECTION('ref_axis',(-1.,0.,0.));
#60674=DIRECTION('',(0.,0.,-1.));
#60675=DIRECTION('center_axis',(0.,0.,-1.));
#60676=DIRECTION('ref_axis',(-1.,0.,0.));
#60677=DIRECTION('center_axis',(0.,0.,-1.));
#60678=DIRECTION('ref_axis',(-1.,0.,0.));
#60679=DIRECTION('',(0.,0.,-1.));
#60680=DIRECTION('center_axis',(0.,0.,-1.));
#60681=DIRECTION('ref_axis',(-1.,0.,0.));
#60682=DIRECTION('',(0.,0.,-1.));
#60683=DIRECTION('center_axis',(0.,0.,-1.));
#60684=DIRECTION('ref_axis',(-1.,0.,0.));
#60685=DIRECTION('center_axis',(0.,0.,-1.));
#60686=DIRECTION('ref_axis',(-1.,0.,0.));
#60687=DIRECTION('',(0.,0.,-1.));
#60688=DIRECTION('center_axis',(0.,0.,-1.));
#60689=DIRECTION('ref_axis',(-1.,0.,0.));
#60690=DIRECTION('',(0.,0.,-1.));
#60691=DIRECTION('center_axis',(0.,0.,-1.));
#60692=DIRECTION('ref_axis',(-1.,0.,0.));
#60693=DIRECTION('center_axis',(0.,0.,-1.));
#60694=DIRECTION('ref_axis',(-1.,0.,0.));
#60695=DIRECTION('',(0.,0.,-1.));
#60696=DIRECTION('center_axis',(0.,0.,-1.));
#60697=DIRECTION('ref_axis',(-1.,0.,0.));
#60698=DIRECTION('',(0.,0.,-1.));
#60699=DIRECTION('center_axis',(0.,0.,-1.));
#60700=DIRECTION('ref_axis',(-1.,0.,0.));
#60701=DIRECTION('center_axis',(0.,0.,-1.));
#60702=DIRECTION('ref_axis',(0.,-1.,0.));
#60703=DIRECTION('',(0.699017620280163,0.715104444495948,0.));
#60704=DIRECTION('',(0.40853671249629,-0.912741888237153,0.));
#60705=DIRECTION('',(0.605841460157257,0.79558539777608,0.));
#60706=DIRECTION('',(0.517605502898811,-0.855619391650791,0.));
#60707=DIRECTION('',(0.503481361059147,0.864006087401026,0.));
#60708=DIRECTION('',(0.618827921495384,-0.785526577257386,0.));
#60709=DIRECTION('',(0.393488997748033,0.919329325460277,0.));
#60710=DIRECTION('',(0.710669539600526,-0.703525980674471,0.));
#60711=DIRECTION('',(0.277531742331645,0.960716468058272,0.));
#60712=DIRECTION('',(0.791738131901976,-0.61086064735942,0.));
#60713=DIRECTION('',(0.157367388601791,0.987540128300948,0.));
#60714=DIRECTION('',(0.860804781177204,-0.508935289307458,0.));
#60715=DIRECTION('',(0.0348175056722151,0.99939368684156,0.));
#60716=DIRECTION('',(0.916822507425865,-0.399294991049663,0.));
#60717=DIRECTION('',(-0.0882601751523597,0.996097455815481,0.));
#60718=DIRECTION('',(0.958942139019354,-0.283601787746457,0.));
#60719=DIRECTION('',(-0.209999921689072,0.977701402725077,0.));
#60720=DIRECTION('',(0.986525185277102,-0.16360947042876,0.));
#60721=DIRECTION('',(-0.328556283475113,0.944484392983294,0.));
#60722=DIRECTION('',(0.999153515334452,-0.0411370003136725,0.));
#60723=DIRECTION('',(-0.442132066915505,0.896949962598262,0.));
#60724=DIRECTION('',(0.996635696580343,0.0819590647934408,0.));
#60725=DIRECTION('',(-0.54900557890607,0.835818685080689,0.));
#60726=DIRECTION('',(0.979009896580564,0.203812714022735,0.));
#60727=DIRECTION('',(-0.647556725945892,0.762017248283946,0.));
#60728=DIRECTION('',(0.946543304496363,0.322576770262686,0.));
#60729=DIRECTION('',(-0.736291573103355,0.676664406760831,0.));
#60730=DIRECTION('',(0.899728080769114,0.436450891482109,0.));
#60731=DIRECTION('',(-0.813864990546873,0.581054022584939,0.));
#60732=DIRECTION('',(0.83927389646971,0.543708862080205,0.));
#60733=DIRECTION('',(-0.879101044341991,0.476635451720516,0.));
#60734=DIRECTION('',(0.766097175408529,0.64272476055546,0.));
#60735=DIRECTION('',(-0.931010822411148,0.364991573263437,0.));
#60736=DIRECTION('',(0.681307202084615,0.731997606818242,0.));
#60737=DIRECTION('',(-0.968807425432727,0.247814794607607,0.));
#60738=DIRECTION('',(0.58618930606342,0.810174115518933,0.));
#60739=DIRECTION('',(-0.991917895432659,0.126881396274019,0.));
#60740=DIRECTION('',(0.482185377690781,0.876069210474377,0.));
#60741=DIRECTION('',(-0.99999190124326,0.00402460530868911,0.));
#60742=DIRECTION('',(0.370872010505059,0.928683989214811,0.));
#60743=DIRECTION('',(-0.992907049166627,-0.118893194570683,0.));
#60744=DIRECTION('',(0.253936601686191,0.967220865327082,0.));
#60745=DIRECTION('',(-0.970770738338343,-0.240008694813393,0.));
#60746=DIRECTION('',(0.13315177283448,0.991095659051655,0.));
#60747=DIRECTION('',(-0.933918532666054,-0.357485907894123,0.));
#60748=DIRECTION('',(0.0103484988340414,0.999946452852292,0.));
#60749=DIRECTION('',(-0.882909074022679,-0.469543999012249,0.));
#60750=DIRECTION('',(-0.112611647860063,0.993639077716975,0.));
#60751=DIRECTION('',(-0.818515613805076,-0.574484281732146,0.));
#60752=DIRECTION('',(-0.233864716762581,0.972269147023373,0.));
#60753=DIRECTION('',(-0.741714291231062,-0.670715968338017,0.));
#60754=DIRECTION('',(-0.351572634947544,0.936160607137494,0.));
#60755=DIRECTION('',(-0.653669336063903,-0.756780284554095,0.));
#60756=DIRECTION('',(-0.463951070360114,0.885860826716988,0.));
#60757=DIRECTION('',(-0.555715420075847,-0.831372583075678,0.));
#60758=DIRECTION('',(-0.569296480471704,0.822132299160257,0.));
#60759=DIRECTION('',(-0.449337424784549,-0.893362120692382,0.));
#60760=DIRECTION('',(-0.666011936248222,0.745941083983778,0.));
#60761=DIRECTION('',(-0.336147932162868,-0.941809199202592,0.));
#60762=DIRECTION('',(-0.752631329966403,0.658442162344578,0.));
#60763=DIRECTION('',(-0.217862779539932,-0.975979410280327,0.));
#60764=DIRECTION('',(-0.827841599912427,0.560961928703217,0.));
#60765=DIRECTION('',(-0.0962750492562598,-0.995354768356843,0.));
#60766=DIRECTION('',(-0.89050263505904,0.45497808403582,0.));
#60767=DIRECTION('',(0.0267721126367755,-0.999641562753852,0.));
#60768=DIRECTION('',(-0.939664557986563,0.342097235393562,0.));
#60769=DIRECTION('',(0.149413436592207,-0.988774810038012,0.));
#60770=DIRECTION('',(-0.974582124056318,0.224030541377457,0.));
#60771=DIRECTION('',(0.269789805152571,-0.962919239103539,0.));
#60772=DIRECTION('',(-0.994726018559695,0.102567772718229,0.));
#60773=DIRECTION('',(0.386076435275407,-0.922466794050081,0.));
#60774=DIRECTION('',(-0.999790880589577,-0.0204498188235966,0.));
#60775=DIRECTION('',(0.496510540184115,-0.868030692709698,0.));
#60776=DIRECTION('',(-0.989699932000427,-0.143157411957434,0.));
#60777=DIRECTION('',(0.599418051418609,-0.800436130889603,0.));
#60778=DIRECTION('',(-0.964606141286711,-0.263694884652627,0.));
#60779=DIRECTION('',(0.693238996006715,-0.720707773244886,0.));
#60780=DIRECTION('',(-0.924889904736447,-0.38023501169225,0.));
#60781=DIRECTION('',(0.77655114406428,-0.63005422040683,0.));
#60782=DIRECTION('',(-0.871153280011235,-0.491011163544849,0.));
#60783=DIRECTION('',(0.848091568350481,-0.529849687829314,0.));
#60784=DIRECTION('',(-0.804210859565811,-0.594344086667328,0.));
#60785=DIRECTION('',(0.906775788957432,-0.421613174083337,0.));
#60786=DIRECTION('',(-0.72507742225678,-0.688667359276932,0.));
#60787=DIRECTION('',(0.951714212920132,-0.306985434387063,0.));
#60788=DIRECTION('',(-0.634952550329563,-0.772551136708751,0.));
#60789=DIRECTION('',(0.982225619539013,-0.187704108429203,0.));
#60790=DIRECTION('',(-0.535202444974341,-0.844723826403333,0.));
#60791=DIRECTION('',(0.997847486991349,-0.0655773795225872,0.));
#60792=DIRECTION('',(-0.427339216108641,-0.904091363953695,0.));
#60793=DIRECTION('',(0.998343003690616,0.0575434356117104,0.));
#60794=DIRECTION('',(-0.312997960332345,-0.949753798006511,0.));
#60795=DIRECTION('',(0.983704658108754,0.179791950918663,0.));
#60796=DIRECTION('',(-0.193911974529963,-0.981018932607262,0.));
#60797=DIRECTION('',(0.954154352643279,0.299315003519512,0.));
#60798=DIRECTION('',(-0.0718864808566897,-0.997412820185324,0.));
#60799=DIRECTION('',(0.910140039803124,0.414300745771919,0.));
#60800=DIRECTION('',(0.0512287385893474,-0.998686946116021,0.));
#60801=DIRECTION('',(0.852328931705225,0.523006111033351,0.));
#60802=DIRECTION('',(0.173567382578051,-0.984821995949017,0.));
#60803=DIRECTION('',(0.781597385818949,0.623783236774591,0.));
#60804=DIRECTION('',(0.293274921971719,-0.956028148195691,0.));
#60805=DIRECTION('center_axis',(0.,0.,-1.));
#60806=DIRECTION('ref_axis',(0.,-1.,0.));
#60807=DIRECTION('',(-0.40853671249629,0.912741888237153,0.));
#60808=DIRECTION('',(-0.699017620280163,-0.715104444495948,0.));
#60809=DIRECTION('',(-0.293274921971719,0.956028148195691,0.));
#60810=DIRECTION('',(-0.781597385818949,-0.623783236774591,0.));
#60811=DIRECTION('',(-0.173567382578051,0.984821995949017,0.));
#60812=DIRECTION('',(-0.852328931705225,-0.523006111033351,0.));
#60813=DIRECTION('',(-0.0512287385893474,0.998686946116021,0.));
#60814=DIRECTION('',(-0.910140039803124,-0.414300745771919,0.));
#60815=DIRECTION('',(0.0718864808566897,0.997412820185324,0.));
#60816=DIRECTION('',(-0.954154352643279,-0.299315003519512,0.));
#60817=DIRECTION('',(0.193911974529963,0.981018932607262,0.));
#60818=DIRECTION('',(-0.983704658108754,-0.179791950918663,0.));
#60819=DIRECTION('',(0.312997960332345,0.949753798006511,0.));
#60820=DIRECTION('',(-0.998343003690616,-0.0575434356117104,0.));
#60821=DIRECTION('',(0.427339216108641,0.904091363953695,0.));
#60822=DIRECTION('',(-0.997847486991349,0.0655773795225872,0.));
#60823=DIRECTION('',(0.535202444974341,0.844723826403333,0.));
#60824=DIRECTION('',(-0.982225619539013,0.187704108429203,0.));
#60825=DIRECTION('',(0.634952550329563,0.772551136708751,0.));
#60826=DIRECTION('',(-0.951714212920132,0.306985434387063,0.));
#60827=DIRECTION('',(0.72507742225678,0.688667359276932,0.));
#60828=DIRECTION('',(-0.906775788957432,0.421613174083337,0.));
#60829=DIRECTION('',(0.804210859565811,0.594344086667328,0.));
#60830=DIRECTION('',(-0.848091568350481,0.529849687829314,0.));
#60831=DIRECTION('',(0.871153280011235,0.491011163544849,0.));
#60832=DIRECTION('',(-0.77655114406428,0.63005422040683,0.));
#60833=DIRECTION('',(0.924889904736447,0.38023501169225,0.));
#60834=DIRECTION('',(-0.693238996006715,0.720707773244886,0.));
#60835=DIRECTION('',(0.964606141286711,0.263694884652627,0.));
#60836=DIRECTION('',(-0.599418051418609,0.800436130889603,0.));
#60837=DIRECTION('',(0.989699932000427,0.143157411957434,0.));
#60838=DIRECTION('',(-0.496510540184115,0.868030692709698,0.));
#60839=DIRECTION('',(0.999790880589577,0.0204498188235966,0.));
#60840=DIRECTION('',(-0.386076435275407,0.922466794050081,0.));
#60841=DIRECTION('',(0.994726018559695,-0.102567772718229,0.));
#60842=DIRECTION('',(-0.269789805152571,0.962919239103539,0.));
#60843=DIRECTION('',(0.974582124056318,-0.224030541377457,0.));
#60844=DIRECTION('',(-0.149413436592207,0.988774810038012,0.));
#60845=DIRECTION('',(0.939664557986563,-0.342097235393562,0.));
#60846=DIRECTION('',(-0.0267721126367755,0.999641562753852,0.));
#60847=DIRECTION('',(0.89050263505904,-0.45497808403582,0.));
#60848=DIRECTION('',(0.0962750492562598,0.995354768356843,0.));
#60849=DIRECTION('',(0.827841599912427,-0.560961928703217,0.));
#60850=DIRECTION('',(0.217862779539932,0.975979410280327,0.));
#60851=DIRECTION('',(0.752631329966403,-0.658442162344578,0.));
#60852=DIRECTION('',(0.336147932162868,0.941809199202592,0.));
#60853=DIRECTION('',(0.666011936248222,-0.745941083983778,0.));
#60854=DIRECTION('',(0.449337424784549,0.893362120692382,0.));
#60855=DIRECTION('',(0.569296480471704,-0.822132299160257,0.));
#60856=DIRECTION('',(0.555715420075847,0.831372583075678,0.));
#60857=DIRECTION('',(0.463951070360114,-0.885860826716988,0.));
#60858=DIRECTION('',(0.653669336063903,0.756780284554095,0.));
#60859=DIRECTION('',(0.351572634947544,-0.936160607137494,0.));
#60860=DIRECTION('',(0.741714291231062,0.670715968338017,0.));
#60861=DIRECTION('',(0.233864716762581,-0.972269147023373,0.));
#60862=DIRECTION('',(0.818515613805076,0.574484281732146,0.));
#60863=DIRECTION('',(0.112611647860063,-0.993639077716975,0.));
#60864=DIRECTION('',(0.88290907402268,0.469543999012249,0.));
#60865=DIRECTION('',(-0.0103484988340414,-0.999946452852292,0.));
#60866=DIRECTION('',(0.933918532666054,0.357485907894123,0.));
#60867=DIRECTION('',(-0.13315177283448,-0.991095659051655,0.));
#60868=DIRECTION('',(0.970770738338343,0.240008694813393,0.));
#60869=DIRECTION('',(-0.253936601686191,-0.967220865327082,0.));
#60870=DIRECTION('',(0.992907049166627,0.118893194570683,0.));
#60871=DIRECTION('',(-0.370872010505059,-0.928683989214811,0.));
#60872=DIRECTION('',(0.99999190124326,-0.00402460530868912,0.));
#60873=DIRECTION('',(-0.482185377690781,-0.876069210474377,0.));
#60874=DIRECTION('',(0.991917895432659,-0.126881396274019,0.));
#60875=DIRECTION('',(-0.58618930606342,-0.810174115518933,0.));
#60876=DIRECTION('',(0.968807425432727,-0.247814794607607,0.));
#60877=DIRECTION('',(-0.681307202084615,-0.731997606818242,0.));
#60878=DIRECTION('',(0.931010822411148,-0.364991573263437,0.));
#60879=DIRECTION('',(-0.766097175408529,-0.64272476055546,0.));
#60880=DIRECTION('',(0.879101044341991,-0.476635451720516,0.));
#60881=DIRECTION('',(-0.83927389646971,-0.543708862080205,0.));
#60882=DIRECTION('',(0.813864990546873,-0.581054022584939,0.));
#60883=DIRECTION('',(-0.899728080769114,-0.436450891482109,0.));
#60884=DIRECTION('',(0.736291573103355,-0.676664406760831,0.));
#60885=DIRECTION('',(-0.946543304496363,-0.322576770262686,0.));
#60886=DIRECTION('',(0.647556725945892,-0.762017248283946,0.));
#60887=DIRECTION('',(-0.979009896580564,-0.203812714022735,0.));
#60888=DIRECTION('',(0.54900557890607,-0.835818685080689,0.));
#60889=DIRECTION('',(-0.996635696580343,-0.0819590647934408,0.));
#60890=DIRECTION('',(0.442132066915505,-0.896949962598262,0.));
#60891=DIRECTION('',(-0.999153515334452,0.0411370003136725,0.));
#60892=DIRECTION('',(0.328556283475113,-0.944484392983294,0.));
#60893=DIRECTION('',(-0.986525185277102,0.16360947042876,0.));
#60894=DIRECTION('',(0.209999921689072,-0.977701402725077,0.));
#60895=DIRECTION('',(-0.958942139019354,0.283601787746457,0.));
#60896=DIRECTION('',(0.0882601751523597,-0.996097455815481,0.));
#60897=DIRECTION('',(-0.916822507425865,0.399294991049663,0.));
#60898=DIRECTION('',(-0.0348175056722151,-0.99939368684156,0.));
#60899=DIRECTION('',(-0.860804781177204,0.508935289307458,0.));
#60900=DIRECTION('',(-0.157367388601791,-0.987540128300948,0.));
#60901=DIRECTION('',(-0.791738131901976,0.61086064735942,0.));
#60902=DIRECTION('',(-0.277531742331645,-0.960716468058272,0.));
#60903=DIRECTION('',(-0.710669539600526,0.703525980674471,0.));
#60904=DIRECTION('',(-0.393488997748033,-0.919329325460277,0.));
#60905=DIRECTION('',(-0.618827921495384,0.785526577257386,0.));
#60906=DIRECTION('',(-0.503481361059147,-0.864006087401026,0.));
#60907=DIRECTION('',(-0.517605502898811,0.855619391650791,0.));
#60908=DIRECTION('',(-0.605841460157257,-0.79558539777608,0.));
#60909=DIRECTION('center_axis',(0.,0.,-1.));
#60910=DIRECTION('ref_axis',(0.,-1.,0.));
#60911=DIRECTION('center_axis',(0.,0.,1.));
#60912=DIRECTION('ref_axis',(1.,0.,0.));
#60913=DIRECTION('center_axis',(0.,0.,1.));
#60914=DIRECTION('ref_axis',(1.,0.,0.));
#60915=DIRECTION('center_axis',(0.,0.,-1.));
#60916=DIRECTION('ref_axis',(0.,-1.,0.));
#60917=DIRECTION('center_axis',(-0.785526577257387,-0.618827921495382,0.));
#60918=DIRECTION('ref_axis',(-0.618827921495382,0.785526577257387,0.));
#60919=DIRECTION('',(0.,0.,-1.));
#60920=DIRECTION('center_axis',(0.864006087401028,-0.503481361059144,0.));
#60921=DIRECTION('ref_axis',(0.,0.,-1.));
#60922=DIRECTION('center_axis',(-0.855619391650793,-0.517605502898808,0.));
#60923=DIRECTION('ref_axis',(-0.517605502898808,0.855619391650792,0.));
#60924=DIRECTION('',(0.,0.,-1.));
#60925=DIRECTION('center_axis',(0.795585397776081,-0.605841460157256,0.));
#60926=DIRECTION('ref_axis',(0.,0.,-1.));
#60927=DIRECTION('center_axis',(-0.703525980674471,-0.710669539600526,0.));
#60928=DIRECTION('ref_axis',(-0.710669539600526,0.703525980674471,0.));
#60929=DIRECTION('',(0.,0.,-1.));
#60930=DIRECTION('center_axis',(0.91932932546028,-0.393488997748027,0.));
#60931=DIRECTION('ref_axis',(0.,0.,-1.));
#60932=DIRECTION('center_axis',(0.203812714022727,-0.979009896580566,0.));
#60933=DIRECTION('ref_axis',(0.,0.,-1.));
#60934=DIRECTION('',(0.,0.,-1.));
#60935=DIRECTION('center_axis',(0.83581868508069,0.549005578906067,0.));
#60936=DIRECTION('ref_axis',(0.,0.,-1.));
#60937=DIRECTION('center_axis',(0.0819590647934317,-0.996635696580343,0.));
#60938=DIRECTION('ref_axis',(0.,0.,-1.));
#60939=DIRECTION('',(0.,0.,-1.));
#60940=DIRECTION('center_axis',(0.896949962598264,0.442132066915501,0.));
#60941=DIRECTION('ref_axis',(0.,0.,-1.));
#60942=DIRECTION('center_axis',(-0.0411370003136629,-0.999153515334452,
0.));
#60943=DIRECTION('ref_axis',(-0.999153515334452,0.0411370003136629,0.));
#60944=DIRECTION('',(0.,0.,-1.));
#60945=DIRECTION('center_axis',(0.944484392983296,0.328556283475108,0.));
#60946=DIRECTION('ref_axis',(0.,0.,-1.));
#60947=DIRECTION('center_axis',(-0.163609470428752,-0.986525185277104,0.));
#60948=DIRECTION('ref_axis',(-0.986525185277104,0.163609470428752,0.));
#60949=DIRECTION('',(0.,0.,-1.));
#60950=DIRECTION('center_axis',(0.977701402725079,0.209999921689065,0.));
#60951=DIRECTION('ref_axis',(0.,0.,-1.));
#60952=DIRECTION('center_axis',(-0.283601787746451,-0.958942139019356,0.));
#60953=DIRECTION('ref_axis',(-0.958942139019356,0.283601787746451,0.));
#60954=DIRECTION('',(0.,0.,-1.));
#60955=DIRECTION('center_axis',(0.996097455815482,0.0882601751523507,0.));
#60956=DIRECTION('ref_axis',(0.,0.,-1.));
#60957=DIRECTION('center_axis',(-0.399294991049658,-0.916822507425867,0.));
#60958=DIRECTION('ref_axis',(-0.916822507425867,0.399294991049658,0.));
#60959=DIRECTION('',(0.,0.,-1.));
#60960=DIRECTION('center_axis',(0.99939368684156,-0.0348175056722054,0.));
#60961=DIRECTION('ref_axis',(0.,0.,-1.));
#60962=DIRECTION('center_axis',(-0.508935289307455,-0.860804781177206,0.));
#60963=DIRECTION('ref_axis',(-0.860804781177206,0.508935289307455,0.));
#60964=DIRECTION('',(0.,0.,-1.));
#60965=DIRECTION('center_axis',(0.98754012830095,-0.157367388601782,0.));
#60966=DIRECTION('ref_axis',(0.,0.,-1.));
#60967=DIRECTION('center_axis',(-0.610860647359419,-0.791738131901977,0.));
#60968=DIRECTION('ref_axis',(-0.791738131901977,0.610860647359419,0.));
#60969=DIRECTION('',(0.,0.,-1.));
#60970=DIRECTION('center_axis',(0.960716468058274,-0.277531742331638,0.));
#60971=DIRECTION('ref_axis',(0.,0.,-1.));
#60972=DIRECTION('center_axis',(0.322576770262681,-0.946543304496365,0.));
#60973=DIRECTION('ref_axis',(0.,0.,-1.));
#60974=DIRECTION('',(0.,0.,-1.));
#60975=DIRECTION('center_axis',(0.762017248283947,0.647556725945891,0.));
#60976=DIRECTION('ref_axis',(0.,0.,-1.));
#60977=DIRECTION('center_axis',(0.436450891482105,-0.899728080769115,0.));
#60978=DIRECTION('ref_axis',(0.,0.,-1.));
#60979=DIRECTION('',(0.,0.,-1.));
#60980=DIRECTION('center_axis',(0.676664406760831,0.736291573103355,0.));
#60981=DIRECTION('ref_axis',(0.,0.,-1.));
#60982=DIRECTION('center_axis',(0.543708862080202,-0.839273896469711,0.));
#60983=DIRECTION('ref_axis',(0.,0.,-1.));
#60984=DIRECTION('',(0.,0.,-1.));
#60985=DIRECTION('center_axis',(0.581054022584937,0.813864990546874,0.));
#60986=DIRECTION('ref_axis',(0.,0.,-1.));
#60987=DIRECTION('center_axis',(0.642724760555459,-0.76609717540853,0.));
#60988=DIRECTION('ref_axis',(0.,0.,-1.));
#60989=DIRECTION('',(0.,0.,-1.));
#60990=DIRECTION('center_axis',(0.476635451720513,0.879101044341993,0.));
#60991=DIRECTION('ref_axis',(0.,0.,-1.));
#60992=DIRECTION('center_axis',(0.731997606818242,-0.681307202084615,0.));
#60993=DIRECTION('ref_axis',(0.,0.,-1.));
#60994=DIRECTION('',(0.,0.,-1.));
#60995=DIRECTION('center_axis',(0.364991573263432,0.93101082241115,0.));
#60996=DIRECTION('ref_axis',(0.,0.,-1.));
#60997=DIRECTION('center_axis',(0.810174115518934,-0.586189306063419,0.));
#60998=DIRECTION('ref_axis',(0.,0.,-1.));
#60999=DIRECTION('',(0.,0.,-1.));
#61000=DIRECTION('center_axis',(0.2478147946076,0.968807425432729,0.));
#61001=DIRECTION('ref_axis',(0.,0.,-1.));
#61002=DIRECTION('center_axis',(0.876069210474379,-0.482185377690778,0.));
#61003=DIRECTION('ref_axis',(0.,0.,-1.));
#61004=DIRECTION('',(0.,0.,-1.));
#61005=DIRECTION('center_axis',(0.12688139627401,0.99191789543266,0.));
#61006=DIRECTION('ref_axis',(0.,0.,-1.));
#61007=DIRECTION('center_axis',(0.928683989214813,-0.370872010505054,0.));
#61008=DIRECTION('ref_axis',(0.,0.,-1.));
#61009=DIRECTION('',(0.,0.,-1.));
#61010=DIRECTION('center_axis',(0.00402460530867915,0.99999190124326,0.));
#61011=DIRECTION('ref_axis',(0.,0.,-1.));
#61012=DIRECTION('center_axis',(0.991095659051657,-0.133151772834472,0.));
#61013=DIRECTION('ref_axis',(0.,0.,-1.));
#61014=DIRECTION('',(0.,0.,-1.));
#61015=DIRECTION('center_axis',(-0.240008694813385,0.970770738338345,0.));
#61016=DIRECTION('ref_axis',(0.,0.,1.));
#61017=DIRECTION('center_axis',(0.967220865327084,-0.253936601686184,0.));
#61018=DIRECTION('ref_axis',(0.,0.,-1.));
#61019=DIRECTION('',(0.,0.,-1.));
#61020=DIRECTION('center_axis',(-0.118893194570674,0.992907049166628,0.));
#61021=DIRECTION('ref_axis',(0.,0.,1.));
#61022=DIRECTION('center_axis',(0.999946452852293,-0.0103484988340315,0.));
#61023=DIRECTION('ref_axis',(0.,0.,-1.));
#61024=DIRECTION('',(0.,0.,-1.));
#61025=DIRECTION('center_axis',(-0.357485907894118,0.933918532666056,0.));
#61026=DIRECTION('ref_axis',(0.,0.,1.));
#61027=DIRECTION('center_axis',(0.993639077716976,0.112611647860054,0.));
#61028=DIRECTION('ref_axis',(0.,0.,-1.));
#61029=DIRECTION('',(0.,0.,-1.));
#61030=DIRECTION('center_axis',(-0.469543999012245,0.882909074022681,0.));
#61031=DIRECTION('ref_axis',(0.,0.,1.));
#61032=DIRECTION('center_axis',(0.972269147023375,0.233864716762574,0.));
#61033=DIRECTION('ref_axis',(0.,0.,-1.));
#61034=DIRECTION('',(0.,0.,-1.));
#61035=DIRECTION('center_axis',(-0.574484281732144,0.818515613805077,0.));
#61036=DIRECTION('ref_axis',(0.,0.,1.));
#61037=DIRECTION('center_axis',(0.936160607137496,0.351572634947539,0.));
#61038=DIRECTION('ref_axis',(0.,0.,-1.));
#61039=DIRECTION('',(0.,0.,-1.));
#61040=DIRECTION('center_axis',(-0.670715968338016,0.741714291231062,0.));
#61041=DIRECTION('ref_axis',(0.,0.,1.));
#61042=DIRECTION('center_axis',(0.88586082671699,0.46395107036011,0.));
#61043=DIRECTION('ref_axis',(0.,0.,-1.));
#61044=DIRECTION('',(0.,0.,-1.));
#61045=DIRECTION('center_axis',(-0.756780284554095,0.653669336063902,0.));
#61046=DIRECTION('ref_axis',(0.,0.,1.));
#61047=DIRECTION('center_axis',(0.822132299160259,0.569296480471702,0.));
#61048=DIRECTION('ref_axis',(0.,0.,-1.));
#61049=DIRECTION('',(0.,0.,-1.));
#61050=DIRECTION('center_axis',(-0.831372583075679,0.555715420075845,0.));
#61051=DIRECTION('ref_axis',(0.,0.,1.));
#61052=DIRECTION('center_axis',(0.745941083983779,0.666011936248222,0.));
#61053=DIRECTION('ref_axis',(0.,0.,-1.));
#61054=DIRECTION('',(0.,0.,-1.));
#61055=DIRECTION('center_axis',(-0.893362120692384,0.449337424784545,0.));
#61056=DIRECTION('ref_axis',(0.,0.,1.));
#61057=DIRECTION('center_axis',(0.658442162344578,0.752631329966403,0.));
#61058=DIRECTION('ref_axis',(0.,0.,-1.));
#61059=DIRECTION('',(0.,0.,-1.));
#61060=DIRECTION('center_axis',(-0.941809199202594,0.336147932162862,0.));
#61061=DIRECTION('ref_axis',(0.,0.,1.));
#61062=DIRECTION('center_axis',(0.560961928703215,0.827841599912429,0.));
#61063=DIRECTION('ref_axis',(0.,0.,-1.));
#61064=DIRECTION('',(0.,0.,-1.));
#61065=DIRECTION('center_axis',(-0.975979410280329,0.217862779539925,0.));
#61066=DIRECTION('ref_axis',(0.,0.,1.));
#61067=DIRECTION('center_axis',(0.454978084035816,0.890502635059042,0.));
#61068=DIRECTION('ref_axis',(0.,0.,-1.));
#61069=DIRECTION('',(0.,0.,-1.));
#61070=DIRECTION('center_axis',(-0.995354768356844,0.0962750492562509,0.));
#61071=DIRECTION('ref_axis',(0.,0.,1.));
#61072=DIRECTION('center_axis',(-0.0204498188235867,0.999790880589577,0.));
#61073=DIRECTION('ref_axis',(0.,0.,1.));
#61074=DIRECTION('',(0.,0.,-1.));
#61075=DIRECTION('center_axis',(-0.922466794050083,-0.386076435275401,0.));
#61076=DIRECTION('ref_axis',(-0.386076435275401,0.922466794050083,0.));
#61077=DIRECTION('center_axis',(0.10256777271822,0.994726018559695,0.));
#61078=DIRECTION('ref_axis',(0.,0.,-1.));
#61079=DIRECTION('',(0.,0.,-1.));
#61080=DIRECTION('center_axis',(-0.96291923910354,-0.269789805152565,0.));
#61081=DIRECTION('ref_axis',(-0.269789805152565,0.96291923910354,0.));
#61082=DIRECTION('center_axis',(0.224030541377449,0.974582124056319,0.));
#61083=DIRECTION('ref_axis',(0.,0.,-1.));
#61084=DIRECTION('',(0.,0.,-1.));
#61085=DIRECTION('center_axis',(-0.988774810038013,-0.149413436592199,0.));
#61086=DIRECTION('ref_axis',(-0.149413436592199,0.988774810038013,0.));
#61087=DIRECTION('center_axis',(0.342097235393556,0.939664557986565,0.));
#61088=DIRECTION('ref_axis',(0.,0.,-1.));
#61089=DIRECTION('',(0.,0.,-1.));
#61090=DIRECTION('center_axis',(-0.999641562753853,-0.0267721126367658,
0.));
#61091=DIRECTION('ref_axis',(-0.0267721126367658,0.999641562753853,0.));
#61092=DIRECTION('center_axis',(-0.143157411957425,0.989699932000428,0.));
#61093=DIRECTION('ref_axis',(0.,0.,1.));
#61094=DIRECTION('',(0.,0.,-1.));
#61095=DIRECTION('center_axis',(-0.8680306927097,-0.496510540184112,0.));
#61096=DIRECTION('ref_axis',(-0.496510540184112,0.8680306927097,0.));
#61097=DIRECTION('center_axis',(-0.26369488465262,0.964606141286713,0.));
#61098=DIRECTION('ref_axis',(0.,0.,1.));
#61099=DIRECTION('',(0.,0.,-1.));
#61100=DIRECTION('center_axis',(-0.800436130889604,-0.599418051418608,0.));
#61101=DIRECTION('ref_axis',(-0.599418051418608,0.800436130889604,0.));
#61102=DIRECTION('center_axis',(-0.380235011692245,0.924889904736449,0.));
#61103=DIRECTION('ref_axis',(0.,0.,1.));
#61104=DIRECTION('',(0.,0.,-1.));
#61105=DIRECTION('center_axis',(-0.720707773244887,-0.693238996006714,0.));
#61106=DIRECTION('ref_axis',(-0.693238996006714,0.720707773244887,0.));
#61107=DIRECTION('center_axis',(-0.491011163544846,0.871153280011237,0.));
#61108=DIRECTION('ref_axis',(0.,0.,1.));
#61109=DIRECTION('',(0.,0.,-1.));
#61110=DIRECTION('center_axis',(-0.630054220406829,-0.776551144064281,0.));
#61111=DIRECTION('ref_axis',(-0.776551144064281,0.630054220406829,0.));
#61112=DIRECTION('center_axis',(-0.594344086667326,0.804210859565812,0.));
#61113=DIRECTION('ref_axis',(0.,0.,1.));
#61114=DIRECTION('',(0.,0.,-1.));
#61115=DIRECTION('center_axis',(-0.529849687829311,-0.848091568350483,0.));
#61116=DIRECTION('ref_axis',(-0.848091568350483,0.529849687829311,0.));
#61117=DIRECTION('center_axis',(-0.688667359276932,0.72507742225678,0.));
#61118=DIRECTION('ref_axis',(0.,0.,1.));
#61119=DIRECTION('',(0.,0.,-1.));
#61120=DIRECTION('center_axis',(-0.421613174083333,-0.906775788957434,0.));
#61121=DIRECTION('ref_axis',(-0.906775788957434,0.421613174083333,0.));
#61122=DIRECTION('center_axis',(-0.772551136708752,0.634952550329562,0.));
#61123=DIRECTION('ref_axis',(0.,0.,1.));
#61124=DIRECTION('',(0.,0.,-1.));
#61125=DIRECTION('center_axis',(-0.306985434387057,-0.951714212920134,0.));
#61126=DIRECTION('ref_axis',(-0.951714212920134,0.306985434387057,0.));
#61127=DIRECTION('center_axis',(-0.844723826403334,0.535202444974339,0.));
#61128=DIRECTION('ref_axis',(0.,0.,1.));
#61129=DIRECTION('',(0.,0.,-1.));
#61130=DIRECTION('center_axis',(-0.187704108429195,-0.982225619539015,0.));
#61131=DIRECTION('ref_axis',(-0.982225619539015,0.187704108429195,0.));
#61132=DIRECTION('center_axis',(-0.904091363953697,0.427339216108637,0.));
#61133=DIRECTION('ref_axis',(0.,0.,1.));
#61134=DIRECTION('',(0.,0.,-1.));
#61135=DIRECTION('center_axis',(-0.0655773795225779,-0.99784748699135,0.));
#61136=DIRECTION('ref_axis',(-0.99784748699135,0.0655773795225779,0.));
#61137=DIRECTION('center_axis',(-0.949753798006513,0.312997960332339,0.));
#61138=DIRECTION('ref_axis',(0.,0.,1.));
#61139=DIRECTION('',(0.,0.,-1.));
#61140=DIRECTION('center_axis',(0.057543435611701,-0.998343003690616,0.));
#61141=DIRECTION('ref_axis',(0.,0.,-1.));
#61142=DIRECTION('center_axis',(-0.981018932607263,0.193911974529956,0.));
#61143=DIRECTION('ref_axis',(0.,0.,1.));
#61144=DIRECTION('',(0.,0.,-1.));
#61145=DIRECTION('center_axis',(0.179791950918655,-0.983704658108756,0.));
#61146=DIRECTION('ref_axis',(0.,0.,-1.));
#61147=DIRECTION('center_axis',(-0.997412820185324,0.0718864808566805,0.));
#61148=DIRECTION('ref_axis',(0.,0.,1.));
#61149=DIRECTION('',(0.,0.,-1.));
#61150=DIRECTION('center_axis',(0.299315003519506,-0.954154352643281,0.));
#61151=DIRECTION('ref_axis',(0.,0.,-1.));
#61152=DIRECTION('center_axis',(-0.998686946116022,-0.051228738589338,0.));
#61153=DIRECTION('ref_axis',(-0.051228738589338,0.998686946116021,0.));
#61154=DIRECTION('',(0.,0.,-1.));
#61155=DIRECTION('center_axis',(0.414300745771915,-0.910140039803126,0.));
#61156=DIRECTION('ref_axis',(0.,0.,-1.));
#61157=DIRECTION('center_axis',(-0.984821995949018,-0.173567382578043,0.));
#61158=DIRECTION('ref_axis',(-0.173567382578043,0.984821995949018,0.));
#61159=DIRECTION('',(0.,0.,-1.));
#61160=DIRECTION('center_axis',(0.523006111033348,-0.852328931705227,0.));
#61161=DIRECTION('ref_axis',(0.,0.,-1.));
#61162=DIRECTION('center_axis',(-0.956028148195693,-0.293274921971712,0.));
#61163=DIRECTION('ref_axis',(-0.293274921971712,0.956028148195693,0.));
#61164=DIRECTION('',(0.,0.,-1.));
#61165=DIRECTION('center_axis',(0.62378323677459,-0.78159738581895,0.));
#61166=DIRECTION('ref_axis',(0.,0.,-1.));
#61167=DIRECTION('center_axis',(-0.912741888237155,-0.408536712496285,0.));
#61168=DIRECTION('ref_axis',(-0.408536712496285,0.912741888237155,0.));
#61169=DIRECTION('',(0.,0.,-1.));
#61170=DIRECTION('center_axis',(0.715104444495948,-0.699017620280163,0.));
#61171=DIRECTION('ref_axis',(0.,0.,-1.));
#106261=CARTESIAN_POINT('',(0.,0.,0.));
#106262=CARTESIAN_POINT('Origin',(-0.00312621780689159,0.00227581852803817,
0.0479362915010152));
#106263=CARTESIAN_POINT('',(-0.0071262178069116,0.00227581852804816,0.05991000000001));
#106264=CARTESIAN_POINT('Origin',(-0.0031262178069016,0.00227581852804816,
0.05991000000001));
#106265=CARTESIAN_POINT('',(-0.0071262178069116,0.00227581852804816,0.05925000000001));
#106266=CARTESIAN_POINT('',(-0.00712621780689159,0.00227581852803817,0.0479362915010152));
#106267=CARTESIAN_POINT('Origin',(-0.0031262178069016,0.00227581852804816,
0.05925000000001));
#106268=CARTESIAN_POINT('Origin',(-0.00312621780689159,0.00227581852803817,
0.06603));
#106269=CARTESIAN_POINT('',(0.0026987821931084,0.00227581852804816,0.06169000000001));
#106270=CARTESIAN_POINT('Origin',(-0.0031262178069016,0.00227581852804816,
0.06169000000001));
#106271=CARTESIAN_POINT('',(0.0026987821931084,0.00227581852804816,0.06603000000001));
#106272=CARTESIAN_POINT('',(0.00269878219310841,0.00227581852803817,0.06603));
#106273=CARTESIAN_POINT('Origin',(-0.0031262178069016,0.00227581852804816,
0.06603000000001));
#106274=CARTESIAN_POINT('Origin',(-0.00312621780689159,0.00227581852803817,
0.06169));
#106275=CARTESIAN_POINT('',(-0.0140012178068916,0.00227581852803817,0.06169000000001));
#106276=CARTESIAN_POINT('Origin',(-0.0031262178069016,0.00227581852804816,
0.06169000000001));
#106277=CARTESIAN_POINT('',(-0.0140012178068916,0.00227581852803817,0.06235000000001));
#106278=CARTESIAN_POINT('',(-0.0140012178068916,0.00227581852803817,0.06169));
#106279=CARTESIAN_POINT('Origin',(-0.0031262178069016,0.00227581852804816,
0.06235000000001));
#106280=CARTESIAN_POINT('Origin',(-0.00312621780689159,0.00227581852803817,
0.05991));
#106281=CARTESIAN_POINT('',(0.00774878219310841,0.00227581852803817,0.05991000000001));
#106282=CARTESIAN_POINT('Origin',(-0.0031262178069016,0.00227581852804816,
0.05991000000001));
#106283=CARTESIAN_POINT('',(0.00774878219310841,0.00227581852803817,0.05925000000001));
#106284=CARTESIAN_POINT('',(0.00774878219310841,0.00227581852803817,0.05991));
#106285=CARTESIAN_POINT('Origin',(-0.0031262178069016,0.00227581852804816,
0.05925000000001));
#106286=CARTESIAN_POINT('Origin',(-0.00312621780689159,0.00227581852803817,
0.06235));
#106287=CARTESIAN_POINT('',(-0.00141627505618096,0.0156670879148174,0.06235));
#106288=CARTESIAN_POINT('',(-0.00141627505618096,0.0156670879148174,0.05925));
#106289=CARTESIAN_POINT('',(-0.00141627505619096,0.0156670879148274,0.0640570798288245));
#106290=CARTESIAN_POINT('',(-0.00173858848307247,0.0157043137847554,0.05925));
#106291=CARTESIAN_POINT('Origin',(-0.0031262178069016,0.00227581852804816,
0.05925000000001));
#106292=CARTESIAN_POINT('',(-0.00173858848307247,0.0157043137847554,0.06235));
#106293=CARTESIAN_POINT('',(-0.00173858848308247,0.0157043137847654,0.0640296944304424));
#106294=CARTESIAN_POINT('Origin',(-0.0031262178069016,0.00227581852804816,
0.06235000000001));
#106295=CARTESIAN_POINT('Origin',(-0.00312621780689159,0.00227581852803817,
0.06235));
#106296=CARTESIAN_POINT('',(-9.89011778140814E-5,0.0154320092391563,0.06235));
#106297=CARTESIAN_POINT('',(-9.89011778140883E-5,0.0154320092391563,0.05925));
#106298=CARTESIAN_POINT('',(-9.89011778240814E-5,0.0154320092391663,0.0640570798288245));
#106299=CARTESIAN_POINT('',(0.000216394654050496,0.0153554569762505,0.06235));
#106300=CARTESIAN_POINT('Origin',(-0.0031262178069016,0.00227581852804816,
0.06235000000001));
#106301=CARTESIAN_POINT('',(0.000216394654050503,0.0153554569762505,0.05925));
#106302=CARTESIAN_POINT('',(0.000216394654060503,0.0153554569762605,0.0640610392221439));
#106303=CARTESIAN_POINT('Origin',(-0.0031262178069016,0.00227581852804816,
0.05925000000001));
#106304=CARTESIAN_POINT('Origin',(-0.00312621780689159,0.00227581852803817,
0.06235));
#106305=CARTESIAN_POINT('',(0.00149489509322412,0.014960270253059,0.06235));
#106306=CARTESIAN_POINT('',(0.00149489509322413,0.014960270253059,0.05925));
#106307=CARTESIAN_POINT('',(0.00149489509323412,0.014960270253069,0.0640610392221439));
#106308=CARTESIAN_POINT('',(0.00179839376664563,0.014845552051458,0.06235));
#106309=CARTESIAN_POINT('Origin',(-0.0031262178069016,0.00227581852804816,
0.06235000000001));
#106310=CARTESIAN_POINT('',(0.00179839376664562,0.014845552051458,0.05925));
#106311=CARTESIAN_POINT('',(0.00179839376665562,0.0148455520514679,0.0640414954613587));
#106312=CARTESIAN_POINT('Origin',(-0.0031262178069016,0.00227581852804816,
0.05925000000001));
#106313=CARTESIAN_POINT('Origin',(-0.00312621780689159,0.00227581852803817,
0.06235));
#106314=CARTESIAN_POINT('',(0.00301864000319971,0.0142962479086285,0.06235));
#106315=CARTESIAN_POINT('',(0.0030186400031997,0.0142962479086285,0.05925));
#106316=CARTESIAN_POINT('',(0.00301864000320971,0.0142962479086385,0.0640414954613587));
#106317=CARTESIAN_POINT('',(0.00330574078765853,0.0141451027793312,0.06235));
#106318=CARTESIAN_POINT('Origin',(-0.0031262178069016,0.00227581852804816,
0.06235000000001));
#106319=CARTESIAN_POINT('',(0.00330574078765853,0.0141451027793312,0.05925));
#106320=CARTESIAN_POINT('',(0.00330574078766853,0.0141451027793412,0.0639988309423612));
#106321=CARTESIAN_POINT('Origin',(-0.0031262178069016,0.00227581852804816,
0.05925000000001));
#106322=CARTESIAN_POINT('Origin',(-0.00312621780689159,0.00227581852803817,
0.06235));
#106323=CARTESIAN_POINT('',(0.00444923513249744,0.0134500081077393,0.06235));
#106324=CARTESIAN_POINT('',(0.00444923513249746,0.0134500081077393,0.05925));
#106325=CARTESIAN_POINT('',(0.00444923513250745,0.0134500081077493,0.0639988309423612));
#106326=CARTESIAN_POINT('',(0.00471558587275565,0.013264727256837,0.06235));
#106327=CARTESIAN_POINT('Origin',(-0.0031262178069016,0.00227581852804816,
0.06235000000001));
#106328=CARTESIAN_POINT('',(0.00471558587275565,0.013264727256837,0.05925));
#106329=CARTESIAN_POINT('',(0.00471558587276565,0.013264727256847,0.0639917959462876));
#106330=CARTESIAN_POINT('Origin',(-0.0031262178069016,0.00227581852804816,
0.05925000000001));
#106331=CARTESIAN_POINT('Origin',(-0.00312621780689159,0.00227581852803817,
0.06235));
#106332=CARTESIAN_POINT('',(0.00576499411722559,0.0124343789831635,0.06235));
#106333=CARTESIAN_POINT('',(0.00576499411722558,0.0124343789831635,0.05925));
#106334=CARTESIAN_POINT('',(0.00576499411723559,0.0124343789831735,0.0639917959462876));
#106335=CARTESIAN_POINT('',(0.00600655720756383,0.012217771079491,0.06235));
#106336=CARTESIAN_POINT('Origin',(-0.0031262178069016,0.00227581852804816,
0.06235000000001));
#106337=CARTESIAN_POINT('',(0.00600655720756383,0.012217771079491,0.05925));
#106338=CARTESIAN_POINT('',(0.00600655720757383,0.012217771079501,0.0640024596936978));
#106339=CARTESIAN_POINT('Origin',(-0.0031262178069016,0.00227581852804816,
0.05925000000001));
#106340=CARTESIAN_POINT('Origin',(-0.00312621780689159,0.00227581852803817,
0.06235));
#106341=CARTESIAN_POINT('',(0.00694597139238648,0.0112647564371543,0.06235));
#106342=CARTESIAN_POINT('',(0.00694597139238648,0.0112647564371543,0.05925));
#106343=CARTESIAN_POINT('',(0.00694597139239648,0.0112647564371643,0.0640024596936978));
#106344=CARTESIAN_POINT('',(0.0071590849825911,0.0110201050357333,0.06235));
#106345=CARTESIAN_POINT('Origin',(-0.0031262178069016,0.00227581852804816,
0.06235000000001));
#106346=CARTESIAN_POINT('',(0.0071590849825911,0.0110201050357333,0.05925));
#106347=CARTESIAN_POINT('',(0.0071590849826011,0.0110201050357433,0.0639889835233611));
#106348=CARTESIAN_POINT('Origin',(-0.0031262178069016,0.00227581852804816,
0.05925000000001));
#106349=CARTESIAN_POINT('Origin',(-0.00312621780689159,0.00227581852803817,
0.06235));
#106350=CARTESIAN_POINT('',(0.00797426454631066,0.00995887075526175,0.06235));
#106351=CARTESIAN_POINT('',(0.00797426454631067,0.00995887075526175,0.05925));
#106352=CARTESIAN_POINT('',(0.00797426454632066,0.00995887075527175,0.0639889835233611));
#106353=CARTESIAN_POINT('',(0.00815569805159019,0.00968988452195386,0.06235));
#106354=CARTESIAN_POINT('Origin',(-0.0031262178069016,0.00227581852804816,
0.06235000000001));
#106355=CARTESIAN_POINT('',(0.00815569805159019,0.00968988452195386,0.05925));
#106356=CARTESIAN_POINT('',(0.00815569805160019,0.00968988452196386,0.0640049766461123));
#106357=CARTESIAN_POINT('Origin',(-0.0031262178069016,0.00227581852804816,
0.05925000000001));
#106358=CARTESIAN_POINT('Origin',(-0.00312621780689159,0.00227581852803817,
0.06235));
#106359=CARTESIAN_POINT('',(0.00883428570296894,0.00853651783327664,0.06235));
#106360=CARTESIAN_POINT('',(0.00883428570296894,0.00853651783327664,0.05925));
#106361=CARTESIAN_POINT('',(0.00883428570297895,0.00853651783328664,0.0640049766461123));
#106362=CARTESIAN_POINT('',(0.00898128877632649,0.00824727432518939,0.06235));
#106363=CARTESIAN_POINT('Origin',(-0.0031262178069016,0.00227581852804816,
0.06235000000001));
#106364=CARTESIAN_POINT('',(0.00898128877632649,0.00824727432518939,0.05925));
#106365=CARTESIAN_POINT('',(0.00898128877633649,0.00824727432519939,0.064044978432889));
#106366=CARTESIAN_POINT('Origin',(-0.0031262178069016,0.00227581852804816,
0.05925000000001));
#106367=CARTESIAN_POINT('Origin',(-0.00312621780689159,0.00227581852803817,
0.06235));
#106368=CARTESIAN_POINT('',(0.00951299781828371,0.00701925909162959,0.06235));
#106369=CARTESIAN_POINT('',(0.0095129978182837,0.00701925909162959,0.05925));
#106370=CARTESIAN_POINT('',(0.00951299781829371,0.00701925909163959,0.064044978432889));
#106371=CARTESIAN_POINT('',(0.00962334204297382,0.00671414294550698,0.06235));
#106372=CARTESIAN_POINT('Origin',(-0.0031262178069016,0.00227581852804816,
0.06235000000001));
#106373=CARTESIAN_POINT('',(0.00962334204297382,0.00671414294550698,0.05925));
#106374=CARTESIAN_POINT('',(0.00962334204298382,0.00671414294551698,0.0640617910186538));
#106375=CARTESIAN_POINT('Origin',(-0.0031262178069016,0.00227581852804816,
0.05925000000001));
#106376=CARTESIAN_POINT('Origin',(-0.00312621780689159,0.00227581852803817,
0.06235));
#106377=CARTESIAN_POINT('',(0.0100001123084278,0.00543009462623556,0.06235));
#106378=CARTESIAN_POINT('',(0.0100001123084278,0.00543009462623556,0.05925));
#106379=CARTESIAN_POINT('',(0.0100001123084378,0.00543009462624556,0.0640617910186538));
#106380=CARTESIAN_POINT('',(0.0100721249784829,0.00511373109183454,0.06235));
#106381=CARTESIAN_POINT('Origin',(-0.0031262178069016,0.00227581852804816,
0.06235000000001));
#106382=CARTESIAN_POINT('',(0.0100721249784829,0.00511373109183452,0.05925));
#106383=CARTESIAN_POINT('',(0.0100721249784929,0.00511373109184452,0.0640550858195668));
#106384=CARTESIAN_POINT('Origin',(-0.0031262178069016,0.00227581852804816,
0.05925000000001));
#106385=CARTESIAN_POINT('Origin',(-0.00312621780689159,0.00227581852803817,
0.06235));
#106386=CARTESIAN_POINT('',(0.0102882450142678,0.00379311455048486,0.06235));
#106387=CARTESIAN_POINT('',(0.0102882450142678,0.00379311455048487,0.05925));
#106388=CARTESIAN_POINT('',(0.0102882450142778,0.00379311455049486,0.0640550858195668));
#106389=CARTESIAN_POINT('',(0.0103208344910155,0.0034702993765037,0.06235));
#106390=CARTESIAN_POINT('Origin',(-0.0031262178069016,0.00227581852804816,
0.06235000000001));
#106391=CARTESIAN_POINT('',(0.0103208344910155,0.0034702993765037,0.05925));
#106392=CARTESIAN_POINT('',(0.0103208344910255,0.0034702993765137,0.0640254477644275));
#106393=CARTESIAN_POINT('Origin',(-0.0031262178069016,0.00227581852804816,
0.05925000000001));
#106394=CARTESIAN_POINT('Origin',(-0.00312621780689159,0.00227581852803817,
0.06235));
#106395=CARTESIAN_POINT('',(0.0103730281376895,0.00213313381368028,0.06235));
#106396=CARTESIAN_POINT('',(0.0103730281376895,0.00213313381368028,0.05925));
#106397=CARTESIAN_POINT('',(0.0103730281376995,0.00213313381369029,0.0640254477644275));
#106398=CARTESIAN_POINT('',(0.0103657003978822,0.00180876054909688,0.06235));
#106399=CARTESIAN_POINT('Origin',(-0.0031262178069016,0.00227581852804816,
0.06235000000001));
#106400=CARTESIAN_POINT('',(0.0103657003978822,0.00180876054909688,0.05925));
#106401=CARTESIAN_POINT('',(0.0103657003978922,0.00180876054910688,0.0640387154811168));
#106402=CARTESIAN_POINT('Origin',(-0.0031262178069016,0.00227581852804816,
0.05925000000001));
#106403=CARTESIAN_POINT('Origin',(-0.00312621780689159,0.00227581852803817,
0.06235));
#106404=CARTESIAN_POINT('',(0.0102531764529649,0.000475316031700583,0.06235));
#106405=CARTESIAN_POINT('',(0.0102531764529649,0.000475316031700583,0.05925));
#106406=CARTESIAN_POINT('',(0.0102531764529749,0.000475316031710583,0.0640387154811168));
#106407=CARTESIAN_POINT('',(0.0102060425776687,0.000154301844558103,0.06235));
#106408=CARTESIAN_POINT('Origin',(-0.0031262178069016,0.00227581852804816,
0.06235000000001));
#106409=CARTESIAN_POINT('',(0.0102060425776687,0.000154301844558114,0.05925));
#106410=CARTESIAN_POINT('',(0.0102060425776787,0.000154301844568114,0.0640602767163006));
#106411=CARTESIAN_POINT('Origin',(-0.0031262178069016,0.00227581852804816,
0.05925000000001));
#106412=CARTESIAN_POINT('Origin',(-0.00312621780689159,0.00227581852803817,
0.06235));
#106413=CARTESIAN_POINT('',(0.00993050678946452,-0.00115520796776584,0.06235));
#106414=CARTESIAN_POINT('',(0.00993050678946452,-0.00115520796776584,0.05925));
#106415=CARTESIAN_POINT('',(0.00993050678947452,-0.00115520796777584,0.0640602767163006));
#106416=CARTESIAN_POINT('',(0.00984428128018315,-0.00146799682961414,0.06235));
#106417=CARTESIAN_POINT('Origin',(-0.0031262178069016,0.00227581852804816,
0.06235000000001));
#106418=CARTESIAN_POINT('',(0.00984428128018315,-0.00146799682961413,0.05925));
#106419=CARTESIAN_POINT('',(0.00984428128019315,-0.00146799682962413,0.06405834964241));
#106420=CARTESIAN_POINT('Origin',(-0.0031262178069016,0.00227581852804816,
0.05925000000001));
#106421=CARTESIAN_POINT('Origin',(-0.00312621780689159,0.00227581852803817,
0.06235));
#106422=CARTESIAN_POINT('',(0.00940991049037555,-0.00273372110295171,0.06235));
#106423=CARTESIAN_POINT('',(0.00940991049037555,-0.0027337211029517,0.05925));
#106424=CARTESIAN_POINT('',(0.00940991049038555,-0.00273372110296171,0.06405834964241));
#106425=CARTESIAN_POINT('',(0.0092859004379363,-0.00303354307919961,0.06235));
#106426=CARTESIAN_POINT('Origin',(-0.0031262178069016,0.00227581852804816,
0.06235000000001));
#106427=CARTESIAN_POINT('',(0.0092859004379363,-0.0030335430791996,0.05925));
#106428=CARTESIAN_POINT('',(0.0092859004379463,-0.0030335430792096,0.064032971803583));
#106429=CARTESIAN_POINT('Origin',(-0.0031262178069016,0.00227581852804816,
0.05925000000001));
#106430=CARTESIAN_POINT('Origin',(-0.00312621780689159,0.00227581852803817,
0.06235));
#106431=CARTESIAN_POINT('',(0.00529718495642217,-0.00827388696012587,0.06235));
#106432=CARTESIAN_POINT('',(0.00529718495642217,-0.00827388696012587,0.05925));
#106433=CARTESIAN_POINT('',(0.00529718495643217,-0.00827388696013587,0.0639818602956537));
#106434=CARTESIAN_POINT('',(0.00554828316999589,-0.00806840849972849,0.05925));
#106435=CARTESIAN_POINT('Origin',(-0.0031262178069016,0.00227581852804816,
0.05925000000001));
#106436=CARTESIAN_POINT('',(0.00554828316999589,-0.00806840849972849,0.06235));
#106437=CARTESIAN_POINT('',(0.00554828317000589,-0.00806840849973849,0.064001351848484));
#106438=CARTESIAN_POINT('Origin',(-0.0031262178069016,0.00227581852804816,
0.06235000000001));
#106439=CARTESIAN_POINT('Origin',(-0.00312621780689159,0.00227581852803817,
0.06235));
#106440=CARTESIAN_POINT('',(0.00652977513110488,-0.00715878800225032,0.06235));
#106441=CARTESIAN_POINT('',(0.00652977513110488,-0.00715878800225032,0.05925));
#106442=CARTESIAN_POINT('',(0.00652977513111488,-0.00715878800226032,0.064001351848484));
#106443=CARTESIAN_POINT('',(0.00675371925143076,-0.00692400993360114,0.05925));
#106444=CARTESIAN_POINT('Origin',(-0.0031262178069016,0.00227581852804816,
0.05925000000001));
#106445=CARTESIAN_POINT('',(0.00675371925143076,-0.00692400993360114,0.06235));
#106446=CARTESIAN_POINT('',(0.00675371925144076,-0.00692400993361114,0.0639967221271783));
#106447=CARTESIAN_POINT('Origin',(-0.0031262178069016,0.00227581852804816,
0.06235000000001));
#106448=CARTESIAN_POINT('Origin',(-0.00312621780689159,0.00227581852803817,
0.06235));
#106449=CARTESIAN_POINT('',(0.00761599029562478,-0.00590067002648398,0.06235));
#106450=CARTESIAN_POINT('',(0.00761599029562478,-0.00590067002648399,0.05925));
#106451=CARTESIAN_POINT('',(0.00761599029563478,-0.00590067002649399,0.0639967221271783));
#106452=CARTESIAN_POINT('',(0.00780938555811477,-0.00564015134578409,0.05925));
#106453=CARTESIAN_POINT('Origin',(-0.0031262178069016,0.00227581852804816,
0.05925000000001));
#106454=CARTESIAN_POINT('',(0.00780938555811477,-0.00564015134578409,0.06235));
#106455=CARTESIAN_POINT('',(0.00780938555812477,-0.00564015134579409,0.0639846412563078));
#106456=CARTESIAN_POINT('Origin',(-0.0031262178069016,0.00227581852804816,
0.06235000000001));
#106457=CARTESIAN_POINT('Origin',(-0.00312621780689159,0.00227581852803817,
0.06235));
#106458=CARTESIAN_POINT('',(0.00869927926492554,-0.00423629472377529,0.06235));
#106459=CARTESIAN_POINT('',(0.00869927926492554,-0.00423629472377528,0.05925));
#106460=CARTESIAN_POINT('',(0.00869927926493554,-0.00423629472378529,0.064032971803583));
#106461=CARTESIAN_POINT('',(0.00853936453531453,-0.00451860481888456,0.06235));
#106462=CARTESIAN_POINT('Origin',(-0.0031262178069016,0.00227581852804816,
0.06235000000001));
#106463=CARTESIAN_POINT('',(0.00853936453531453,-0.00451860481888456,0.05925));
#106464=CARTESIAN_POINT('',(0.00853936453532453,-0.00451860481889456,0.0639846412563078));
#106465=CARTESIAN_POINT('Origin',(-0.0031262178069016,0.00227581852804816,
0.05925000000001));
#106466=CARTESIAN_POINT('Origin',(-0.00312621780689159,0.00227581852803817,
0.06235));
#106467=CARTESIAN_POINT('',(0.0042113504960508,-0.00905599912843934,0.06235));
#106468=CARTESIAN_POINT('',(0.0042113504960508,-0.00905599912843933,0.05925));
#106469=CARTESIAN_POINT('',(0.00421135049606079,-0.00905599912844934,0.0639818602956537));
#106470=CARTESIAN_POINT('',(0.00393690458219163,-0.00922906313657846,0.06235));
#106471=CARTESIAN_POINT('Origin',(-0.0031262178069016,0.00227581852804816,
0.06235000000001));
#106472=CARTESIAN_POINT('',(0.00393690458219163,-0.00922906313657845,0.05925));
#106473=CARTESIAN_POINT('',(0.00393690458220163,-0.00922906313658845,0.0640171157235625));
#106474=CARTESIAN_POINT('Origin',(-0.0031262178069016,0.00227581852804816,
0.05925000000001));
#106475=CARTESIAN_POINT('Origin',(-0.00312621780689159,0.00227581852803817,
0.06235));
#106476=CARTESIAN_POINT('',(0.00276318776613839,-0.00987181095249685,0.06235));
#106477=CARTESIAN_POINT('',(0.00276318776613839,-0.00987181095249684,0.05925));
#106478=CARTESIAN_POINT('',(0.0027631877661484,-0.00987181095250685,0.0640171157235625));
#106479=CARTESIAN_POINT('',(0.00246955447229308,-0.0100098370344261,0.06235));
#106480=CARTESIAN_POINT('Origin',(-0.0031262178069016,0.00227581852804816,
0.06235000000001));
#106481=CARTESIAN_POINT('',(0.00246955447229308,-0.0100098370344261,0.05925));
#106482=CARTESIAN_POINT('',(0.00246955447230308,-0.0100098370344361,0.0640513762773574));
#106483=CARTESIAN_POINT('Origin',(-0.0031262178069016,0.00227581852804816,
0.05925000000001));
#106484=CARTESIAN_POINT('Origin',(-0.00312621780689159,0.00227581852803817,
0.06235));
#106485=CARTESIAN_POINT('',(0.00122574765106832,-0.0105034770962411,0.06235));
#106486=CARTESIAN_POINT('',(0.00122574765106833,-0.0105034770962411,0.05925));
#106487=CARTESIAN_POINT('',(0.00122574765107832,-0.0105034770962511,0.0640513762773574));
#106488=CARTESIAN_POINT('',(0.00091737815865827,-0.0106043729172544,0.06235));
#106489=CARTESIAN_POINT('Origin',(-0.0031262178069016,0.00227581852804816,
0.06235000000001));
#106490=CARTESIAN_POINT('',(0.00091737815865827,-0.0106043729172544,0.05925));
#106491=CARTESIAN_POINT('',(0.00091737815866827,-0.0106043729172644,0.0640623222440636));
#106492=CARTESIAN_POINT('Origin',(-0.0031262178069016,0.00227581852804816,
0.05925000000001));
#106493=CARTESIAN_POINT('Origin',(-0.00312621780689159,0.00227581852803817,
0.06235));
#106494=CARTESIAN_POINT('',(-0.000377663824195094,-0.010941422144818,0.06235));
#106495=CARTESIAN_POINT('',(-0.000377663824195087,-0.010941422144818,0.05925));
#106496=CARTESIAN_POINT('',(-0.000377663824205095,-0.010941422144828,0.0640623222440636));
#106497=CARTESIAN_POINT('',(-0.000696094947999507,-0.0110036582271164,0.06235));
#106498=CARTESIAN_POINT('Origin',(-0.0031262178069016,0.00227581852804816,
0.06235000000001));
#106499=CARTESIAN_POINT('',(-0.000696094947999507,-0.0110036582271164,0.05925));
#106500=CARTESIAN_POINT('',(-0.000696094948009507,-0.0110036582271264,0.0640497400911727));
#106501=CARTESIAN_POINT('Origin',(-0.0031262178069016,0.00227581852804816,
0.05925000000001));
#106502=CARTESIAN_POINT('Origin',(-0.00312621780689159,0.00227581852803817,
0.06235));
#106503=CARTESIAN_POINT('',(-0.00202274057611456,-0.0111790072977077,0.06235));
#106504=CARTESIAN_POINT('',(-0.00202274057611456,-0.0111790072977077,0.05925));
#106505=CARTESIAN_POINT('',(-0.00202274057612456,-0.0111790072977176,0.0640497400911727));
#106506=CARTESIAN_POINT('',(-0.00234640624006724,-0.0112016402057234,0.06235));
#106507=CARTESIAN_POINT('Origin',(-0.0031262178069016,0.00227581852804816,
0.06235000000001));
#106508=CARTESIAN_POINT('',(-0.00234640624006724,-0.0112016402057234,0.05925));
#106509=CARTESIAN_POINT('',(-0.00234640624007724,-0.0112016402057334,0.0640207658501784));
#106510=CARTESIAN_POINT('Origin',(-0.0031262178069016,0.00227581852804816,
0.05925000000001));
#106511=CARTESIAN_POINT('Origin',(-0.00312621780689159,0.00227581852803817,
0.06235));
#106512=CARTESIAN_POINT('',(-0.00368454491802983,-0.0112126310061732,0.06235));
#106513=CARTESIAN_POINT('',(-0.00368454491802983,-0.0112126310061732,0.05925));
#106514=CARTESIAN_POINT('',(-0.00368454491803983,-0.0112126310061832,0.0640207658501784));
#106515=CARTESIAN_POINT('',(-0.00400853868059187,-0.0111953176480916,0.06235));
#106516=CARTESIAN_POINT('Origin',(-0.0031262178069016,0.00227581852804816,
0.06235000000001));
#106517=CARTESIAN_POINT('',(-0.00400853868059187,-0.0111953176480916,0.05925));
#106518=CARTESIAN_POINT('',(-0.00400853868060188,-0.0111953176481016,0.0640462926264831));
#106519=CARTESIAN_POINT('Origin',(-0.0031262178069016,0.00227581852804816,
0.05925000000001));
#106520=CARTESIAN_POINT('Origin',(-0.00312621780689159,0.00227581852803817,
0.06235));
#106521=CARTESIAN_POINT('',(-0.00533788559006755,-0.0110417835690686,0.06235));
#106522=CARTESIAN_POINT('',(-0.00533788559006755,-0.0110417835690686,0.05925));
#106523=CARTESIAN_POINT('',(-0.00533788559007755,-0.0110417835690786,0.0640462926264831));
#106524=CARTESIAN_POINT('',(-0.00565729603605961,-0.0109847863977498,0.06235));
#106525=CARTESIAN_POINT('Origin',(-0.0031262178069016,0.00227581852804816,
0.06235000000001));
#106526=CARTESIAN_POINT('',(-0.00565729603605961,-0.0109847863977498,0.05925));
#106527=CARTESIAN_POINT('',(-0.00565729603606961,-0.0109847863977598,0.0640620033446139));
#106528=CARTESIAN_POINT('Origin',(-0.0031262178069016,0.00227581852804816,
0.05925000000001));
#106529=CARTESIAN_POINT('Origin',(-0.00312621780689159,0.00227581852803817,
0.06235));
#106530=CARTESIAN_POINT('',(-0.00695769963296234,-0.0106690548593878,0.06235));
#106531=CARTESIAN_POINT('',(-0.00695769963296234,-0.0106690548593878,0.05925));
#106532=CARTESIAN_POINT('',(-0.00695769963297234,-0.0106690548593978,0.0640620033446139));
#106533=CARTESIAN_POINT('',(-0.00726768482561223,-0.0105732378938494,0.06235));
#106534=CARTESIAN_POINT('Origin',(-0.0031262178069016,0.00227581852804816,
0.06235000000001));
#106535=CARTESIAN_POINT('',(-0.00726768482561223,-0.0105732378938494,0.05925));
#106536=CARTESIAN_POINT('',(-0.00726768482562223,-0.0105732378938594,0.0640541921468464));
#106537=CARTESIAN_POINT('Origin',(-0.0031262178069016,0.00227581852804816,
0.05925000000001));
#106538=CARTESIAN_POINT('Origin',(-0.00312621780689159,0.00227581852803817,
0.06235));
#106539=CARTESIAN_POINT('',(-0.00851943231697142,-0.0101000950644311,0.06235));
#106540=CARTESIAN_POINT('',(-0.00851943231697142,-0.010100095064431,0.05925));
#106541=CARTESIAN_POINT('',(-0.00851943231698142,-0.0101000950644411,0.0640541921468464));
#106542=CARTESIAN_POINT('',(-0.00881529319674008,-0.00996691079220006,0.06235));
#106543=CARTESIAN_POINT('Origin',(-0.0031262178069016,0.00227581852804816,
0.06235000000001));
#106544=CARTESIAN_POINT('',(-0.00881529319674006,-0.00996691079220006,0.05925));
#106545=CARTESIAN_POINT('',(-0.00881529319675006,-0.00996691079221006,0.064023011312257));
#106546=CARTESIAN_POINT('Origin',(-0.0031262178069016,0.00227581852804816,
0.05925000000001));
#106547=CARTESIAN_POINT('Origin',(-0.00312621780689159,0.00227581852803817,
0.06235));
#106548=CARTESIAN_POINT('',(-0.00999940936654784,-0.00934352903472414,0.06235));
#106549=CARTESIAN_POINT('',(-0.00999940936654784,-0.00934352903472414,0.05925));
#106550=CARTESIAN_POINT('',(-0.00999940936655784,-0.00934352903473414,0.064023011312257));
#106551=CARTESIAN_POINT('',(-0.0102766609840819,-0.00917499639360702,0.06235));
#106552=CARTESIAN_POINT('Origin',(-0.0031262178069016,0.00227581852804816,
0.06235000000001));
#106553=CARTESIAN_POINT('',(-0.0102766609840819,-0.00917499639360702,0.05925));
#106554=CARTESIAN_POINT('',(-0.0102766609840919,-0.00917499639361702,0.0639774518569539));
#106555=CARTESIAN_POINT('Origin',(-0.0031262178069016,0.00227581852804816,
0.05925000000001));
#106556=CARTESIAN_POINT('Origin',(-0.00312621780689159,0.00227581852803817,
0.06235));
#106557=CARTESIAN_POINT('',(-0.0128537065572342,-0.00708505550230524,0.06235));
#106558=CARTESIAN_POINT('',(-0.0128537065572342,-0.00708505550230524,0.05925));
#106559=CARTESIAN_POINT('',(-0.0128537065572442,-0.00708505550231524,0.0639987344374706));
#106560=CARTESIAN_POINT('',(-0.0126259362114935,-0.00731612341472131,0.05925));
#106561=CARTESIAN_POINT('Origin',(-0.0031262178069016,0.00227581852804816,
0.05925000000001));
#106562=CARTESIAN_POINT('',(-0.0126259362114935,-0.00731612341472131,0.06235));
#106563=CARTESIAN_POINT('',(-0.0126259362115035,-0.00731612341473131,0.0640001436149048));
#106564=CARTESIAN_POINT('Origin',(-0.0031262178069016,0.00227581852804816,
0.06235000000001));
#106565=CARTESIAN_POINT('Origin',(-0.00312621780689159,0.00227581852803817,
0.06235));
#106566=CARTESIAN_POINT('',(-0.0113751958382256,-0.00841082554007646,0.06235));
#106567=CARTESIAN_POINT('',(-0.0113751958382256,-0.00841082554007647,0.05925));
#106568=CARTESIAN_POINT('',(-0.0113751958382356,-0.00841082554008646,0.0639774518569539));
#106569=CARTESIAN_POINT('',(-0.011629635341618,-0.00820949931311987,0.06235));
#106570=CARTESIAN_POINT('Origin',(-0.0031262178069016,0.00227581852804816,
0.06235000000001));
#106571=CARTESIAN_POINT('',(-0.011629635341618,-0.00820949931311987,0.05925));
#106572=CARTESIAN_POINT('',(-0.011629635341628,-0.00820949931312987,0.0640001436149048));
#106573=CARTESIAN_POINT('Origin',(-0.0031262178069016,0.00227581852804816,
0.05925000000001));
#106574=CARTESIAN_POINT('Origin',(-0.00312621780689159,0.00227581852803817,
0.06235));
#106575=CARTESIAN_POINT('',(-0.0137326705372273,-0.00607601722700116,0.06235));
#106576=CARTESIAN_POINT('',(-0.0137326705372273,-0.00607601722700116,0.05925));
#106577=CARTESIAN_POINT('',(-0.0137326705372373,-0.00607601722701116,0.0639987344374706));
#106578=CARTESIAN_POINT('',(-0.0139303189590513,-0.00581871038314018,0.06235));
#106579=CARTESIAN_POINT('Origin',(-0.0031262178069016,0.00227581852804816,
0.06235000000001));
#106580=CARTESIAN_POINT('',(-0.0139303189590513,-0.00581871038314018,0.05925));
#106581=CARTESIAN_POINT('',(-0.0139303189590613,-0.00581871038315018,0.06397650941056));
#106582=CARTESIAN_POINT('Origin',(-0.0031262178069016,0.00227581852804816,
0.05925000000001));
#106583=CARTESIAN_POINT('Origin',(-0.00312621780689159,0.00227581852803817,
0.06235));
#106584=CARTESIAN_POINT('',(-0.0146786218511919,-0.00470930572262721,0.06235));
#106585=CARTESIAN_POINT('',(-0.0146786218511919,-0.00470930572262721,0.05925));
#106586=CARTESIAN_POINT('',(-0.0146786218512019,-0.00470930572263721,0.06397650941056));
#106587=CARTESIAN_POINT('',(-0.0148431522004959,-0.00442966045679009,0.06235));
#106588=CARTESIAN_POINT('Origin',(-0.0031262178069016,0.00227581852804816,
0.06235000000001));
#106589=CARTESIAN_POINT('',(-0.0148431522004959,-0.00442966045679009,0.05925));
#106590=CARTESIAN_POINT('',(-0.0148431522005059,-0.00442966045680008,0.0640278376069454));
#106591=CARTESIAN_POINT('Origin',(-0.0031262178069016,0.00227581852804816,
0.05925000000001));
#106592=CARTESIAN_POINT('Origin',(-0.00312621780689159,0.00227581852803817,
0.06235));
#106593=CARTESIAN_POINT('',(-0.0154494504957172,-0.00323670685485675,0.06235));
#106594=CARTESIAN_POINT('',(-0.0154494504957172,-0.00323670685485676,0.05925));
#106595=CARTESIAN_POINT('',(-0.0154494504957272,-0.00323670685486675,0.0640278376069454));
#106596=CARTESIAN_POINT('',(-0.0155783686601187,-0.00293896230421893,0.06235));
#106597=CARTESIAN_POINT('Origin',(-0.0031262178069016,0.00227581852804816,
0.06235000000001));
#106598=CARTESIAN_POINT('',(-0.0155783686601187,-0.00293896230421893,0.05925));
#106599=CARTESIAN_POINT('',(-0.0155783686601287,-0.00293896230422892,0.0640563147052341));
#106600=CARTESIAN_POINT('Origin',(-0.0031262178069016,0.00227581852804816,
0.05925000000001));
#106601=CARTESIAN_POINT('Origin',(-0.00312621780689159,0.00227581852803817,
0.06235));
#106602=CARTESIAN_POINT('',(-0.0160334714942915,-0.00168054372144059,0.06235));
#106603=CARTESIAN_POINT('',(-0.0160334714942915,-0.00168054372144059,0.05925));
#106604=CARTESIAN_POINT('',(-0.0160334714943015,-0.00168054372145059,0.0640563147052341));
#106605=CARTESIAN_POINT('',(-0.0161248232058302,-0.00136921338988561,0.06235));
#106606=CARTESIAN_POINT('Origin',(-0.0031262178069016,0.00227581852804816,
0.06235000000001));
#106607=CARTESIAN_POINT('',(-0.0161248232058302,-0.00136921338988561,0.05925));
#106608=CARTESIAN_POINT('',(-0.0161248232058402,-0.00136921338989561,0.064061380725474));
#106609=CARTESIAN_POINT('Origin',(-0.0031262178069016,0.00227581852804816,
0.05925000000001));
#106610=CARTESIAN_POINT('Origin',(-0.00312621780689159,0.00227581852803817,
0.06235));
#106611=CARTESIAN_POINT('',(-0.0164218316838949,-6.44061692159324E-5,0.06235));
#106612=CARTESIAN_POINT('',(-0.0164218316838948,-6.44061692159359E-5,0.05925));
#106613=CARTESIAN_POINT('',(-0.0164218316839049,-6.44061692259324E-5,0.064061380725474));
#106614=CARTESIAN_POINT('',(-0.0164742321437426,0.000255790492782481,0.06235));
#106615=CARTESIAN_POINT('Origin',(-0.0031262178069016,0.00227581852804816,
0.06235000000001));
#106616=CARTESIAN_POINT('',(-0.0164742321437426,0.000255790492782477,0.05925));
#106617=CARTESIAN_POINT('',(-0.0164742321437527,0.000255790492792477,0.0640429369448856));
#106618=CARTESIAN_POINT('Origin',(-0.0031262178069016,0.00227581852804816,
0.05925000000001));
#106619=CARTESIAN_POINT('Origin',(-0.00312621780689159,0.00227581852803817,
0.06235));
#106620=CARTESIAN_POINT('',(-0.0166086439199253,0.00158720680392539,0.06235));
#106621=CARTESIAN_POINT('',(-0.0166086439199253,0.00158720680392539,0.05925));
#106622=CARTESIAN_POINT('',(-0.0166086439199353,0.00158720680393539,0.0640429369448856));
#106623=CARTESIAN_POINT('',(-0.016621298790525,0.00191141594136183,0.06235));
#106624=CARTESIAN_POINT('Origin',(-0.0031262178069016,0.00227581852804816,
0.06235000000001));
#106625=CARTESIAN_POINT('',(-0.016621298790525,0.00191141594136184,0.05925));
#106626=CARTESIAN_POINT('',(-0.016621298790535,0.00191141594137184,0.0640221869975759));
#106627=CARTESIAN_POINT('Origin',(-0.0031262178069016,0.00227581852804816,
0.05925000000001));
#106628=CARTESIAN_POINT('Origin',(-0.00312621780689159,0.00227581852803817,
0.06235));
#106629=CARTESIAN_POINT('',(-0.0165910763193107,0.00324925842887212,0.06235));
#106630=CARTESIAN_POINT('',(-0.0165910763193107,0.00324925842887211,0.05925));
#106631=CARTESIAN_POINT('',(-0.0165910763193207,0.00324925842888212,0.0640221869975759));
#106632=CARTESIAN_POINT('',(-0.0165637937657236,0.00357256536170368,0.06235));
#106633=CARTESIAN_POINT('Origin',(-0.0031262178069016,0.00227581852804816,
0.06235000000001));
#106634=CARTESIAN_POINT('',(-0.0165637937657236,0.00357256536170368,0.05925));
#106635=CARTESIAN_POINT('',(-0.0165637937657335,0.00357256536171368,0.0640524165708933));
#106636=CARTESIAN_POINT('Origin',(-0.0031262178069016,0.00227581852804816,
0.05925000000001));
#106637=CARTESIAN_POINT('Origin',(-0.00312621780689159,0.00227581852803817,
0.06235));
#106638=CARTESIAN_POINT('',(-0.0163693951889687,0.00489655369719221,0.06235));
#106639=CARTESIAN_POINT('',(-0.0163693951889687,0.00489655369719221,0.05925));
#106640=CARTESIAN_POINT('',(-0.0163693951889787,0.00489655369720221,0.0640524165708933));
#106641=CARTESIAN_POINT('',(-0.0163025887868969,0.00521405742187809,0.06235));
#106642=CARTESIAN_POINT('Origin',(-0.0031262178069016,0.00227581852804816,
0.06235000000001));
#106643=CARTESIAN_POINT('',(-0.0163025887868969,0.00521405742187809,0.05925));
#106644=CARTESIAN_POINT('',(-0.0163025887869069,0.00521405742188809,0.0640622576161447));
#106645=CARTESIAN_POINT('Origin',(-0.0031262178069016,0.00227581852804816,
0.05925000000001));
#106646=CARTESIAN_POINT('Origin',(-0.00312621780689159,0.00227581852803817,
0.06235));
#106647=CARTESIAN_POINT('',(-0.00795506065672538,0.0148826530526763,0.06235));
#106648=CARTESIAN_POINT('',(-0.00795506065672538,0.0148826530526763,0.05925));
#106649=CARTESIAN_POINT('',(-0.00795506065673538,0.0148826530526863,0.0640597876943085));
#106650=CARTESIAN_POINT('',(-0.0082566340354141,0.0147629650924905,0.05925));
#106651=CARTESIAN_POINT('Origin',(-0.0031262178069016,0.00227581852804816,
0.05925000000001));
#106652=CARTESIAN_POINT('',(-0.0082566340354141,0.0147629650924905,0.06235));
#106653=CARTESIAN_POINT('',(-0.0082566340354241,0.0147629650925005,0.0640371289970171));
#106654=CARTESIAN_POINT('Origin',(-0.0031262178069016,0.00227581852804816,
0.06235000000001));
#106655=CARTESIAN_POINT('Origin',(-0.00312621780689159,0.00227581852803817,
0.06235));
#106656=CARTESIAN_POINT('',(-0.00946769283447502,0.0141936914286247,0.06235));
#106657=CARTESIAN_POINT('',(-0.00946769283447502,0.0141936914286247,0.05925));
#106658=CARTESIAN_POINT('',(-0.00946769283448502,0.0141936914286347,0.0640371289970171));
#106659=CARTESIAN_POINT('',(-0.00975227219181637,0.0140378508051584,0.05925));
#106660=CARTESIAN_POINT('Origin',(-0.0031262178069016,0.00227581852804816,
0.05925000000001));
#106661=CARTESIAN_POINT('',(-0.00975227219181637,0.0140378508051584,0.06235));
#106662=CARTESIAN_POINT('',(-0.00975227219182637,0.0140378508051684,0.0639914355303226));
#106663=CARTESIAN_POINT('Origin',(-0.0031262178069016,0.00227581852804816,
0.06235000000001));
#106664=CARTESIAN_POINT('Origin',(-0.00312621780689159,0.00227581852803817,
0.06235));
#106665=CARTESIAN_POINT('',(-0.0108841947149502,0.0133240669998109,0.06235));
#106666=CARTESIAN_POINT('',(-0.0108841947149502,0.0133240669998109,0.05925));
#106667=CARTESIAN_POINT('',(-0.0108841947149602,0.0133240669998209,0.0639914355303226));
#106668=CARTESIAN_POINT('',(-0.0111474661179711,0.0131344360980608,0.05925));
#106669=CARTESIAN_POINT('Origin',(-0.0031262178069016,0.00227581852804816,
0.05925000000001));
#106670=CARTESIAN_POINT('',(-0.0111474661179711,0.0131344360980608,0.06235));
#106671=CARTESIAN_POINT('',(-0.0111474661179811,0.0131344360980708,0.0639946102147355));
#106672=CARTESIAN_POINT('Origin',(-0.0031262178069016,0.00227581852804816,
0.06235000000001));
#106673=CARTESIAN_POINT('Origin',(-0.00312621780689159,0.00227581852803817,
0.06235));
#106674=CARTESIAN_POINT('',(-0.0121830935735454,0.0122869623861294,0.06235));
#106675=CARTESIAN_POINT('',(-0.0121830935735454,0.0122869623861294,0.05925));
#106676=CARTESIAN_POINT('',(-0.0121830935735554,0.0122869623861394,0.0639946102147355));
#106677=CARTESIAN_POINT('',(-0.0124210660961402,0.0120664158172669,0.05925));
#106678=CARTESIAN_POINT('Origin',(-0.0031262178069016,0.00227581852804816,
0.05925000000001));
#106679=CARTESIAN_POINT('',(-0.0124210660961402,0.0120664158172669,0.06235));
#106680=CARTESIAN_POINT('',(-0.0124210660961502,0.0120664158172769,0.0640020568079385));
#106681=CARTESIAN_POINT('Origin',(-0.0031262178069016,0.00227581852804816,
0.06235000000001));
#106682=CARTESIAN_POINT('Origin',(-0.00312621780689159,0.00227581852803817,
0.06235));
#106683=CARTESIAN_POINT('',(-0.013344699427589,0.0110980990363574,0.06235));
#106684=CARTESIAN_POINT('',(-0.013344699427589,0.0110980990363574,0.05925));
#106685=CARTESIAN_POINT('',(-0.013344699427599,0.0110980990363674,0.0640020568079385));
#106686=CARTESIAN_POINT('',(-0.0135537656488909,0.0108499800615536,0.05925));
#106687=CARTESIAN_POINT('Origin',(-0.0031262178069016,0.00227581852804816,
0.05925000000001));
#106688=CARTESIAN_POINT('',(-0.0135537656488909,0.0108499800615536,0.06235));
#106689=CARTESIAN_POINT('',(-0.0135537656489009,0.0108499800615636,0.0639853702628634));
#106690=CARTESIAN_POINT('Origin',(-0.0031262178069016,0.00227581852804816,
0.06235000000001));
#106691=CARTESIAN_POINT('Origin',(-0.00312621780689159,0.00227581852803817,
0.06235));
#106692=CARTESIAN_POINT('',(-0.0143514035164094,0.00977549890701684,0.06235));
#106693=CARTESIAN_POINT('',(-0.0143514035164094,0.00977549890701684,0.05925));
#106694=CARTESIAN_POINT('',(-0.0143514035164194,0.00977549890702684,0.0639853702628634));
#106695=CARTESIAN_POINT('',(-0.0145283942056139,0.0095035687570112,0.05925));
#106696=CARTESIAN_POINT('Origin',(-0.0031262178069016,0.00227581852804816,
0.05925000000001));
#106697=CARTESIAN_POINT('',(-0.0145283942056139,0.00950356875701119,0.06235));
#106698=CARTESIAN_POINT('',(-0.0145283942056239,0.00950356875702119,0.0640116263041442));
#106699=CARTESIAN_POINT('Origin',(-0.0031262178069016,0.00227581852804816,
0.06235000000001));
#106700=CARTESIAN_POINT('Origin',(-0.00312621780689159,0.00227581852803817,
0.06235));
#106701=CARTESIAN_POINT('',(-0.0151879452321978,0.00833921126788417,0.06235));
#106702=CARTESIAN_POINT('',(-0.0151879452321978,0.00833921126788417,0.05925));
#106703=CARTESIAN_POINT('',(-0.0151879452322077,0.00833921126789417,0.0640116263041442));
#106704=CARTESIAN_POINT('',(-0.0153301773908709,0.0080475921265605,0.05925));
#106705=CARTESIAN_POINT('Origin',(-0.0031262178069016,0.00227581852804816,
0.05925000000001));
#106706=CARTESIAN_POINT('',(-0.0153301773908709,0.0080475921265605,0.06235));
#106707=CARTESIAN_POINT('',(-0.0153301773908809,0.0080475921265705,0.0640485717989525));
#106708=CARTESIAN_POINT('Origin',(-0.0031262178069016,0.00227581852804816,
0.06235000000001));
#106709=CARTESIAN_POINT('Origin',(-0.00312621780689159,0.00227581852803817,
0.06235));
#106710=CARTESIAN_POINT('',(-0.0159469609888662,0.00650412129177826,0.06235));
#106711=CARTESIAN_POINT('',(-0.0159469609888662,0.00650412129177825,0.05925));
#106712=CARTESIAN_POINT('',(-0.0159469609888762,0.00650412129178826,0.0640622576161447));
#106713=CARTESIAN_POINT('',(-0.0158416434552664,0.00681100877549768,0.06235));
#106714=CARTESIAN_POINT('Origin',(-0.0031262178069016,0.00227581852804816,
0.06235000000001));
#106715=CARTESIAN_POINT('',(-0.0158416434552664,0.00681100877549768,0.05925));
#106716=CARTESIAN_POINT('',(-0.0158416434552764,0.00681100877550768,0.0640485717989525));
#106717=CARTESIAN_POINT('Origin',(-0.0031262178069016,0.00227581852804816,
0.05925000000001));
#106718=CARTESIAN_POINT('Origin',(-0.00312621780689159,0.00227581852803817,
0.06235));
#106719=CARTESIAN_POINT('',(-0.00668322399864577,0.0152987869666017,0.06235));
#106720=CARTESIAN_POINT('',(-0.00668322399864577,0.0152987869666017,0.05925));
#106721=CARTESIAN_POINT('',(-0.00668322399865577,0.0152987869666117,0.0640597876943085));
#106722=CARTESIAN_POINT('',(-0.00636922814362363,0.0153805079160339,0.06235));
#106723=CARTESIAN_POINT('Origin',(-0.0031262178069016,0.00227581852804816,
0.06235000000001));
#106724=CARTESIAN_POINT('',(-0.00636922814362363,0.0153805079160339,0.05925));
#106725=CARTESIAN_POINT('',(-0.00636922814363363,0.015380507916044,0.0640589676062857));
#106726=CARTESIAN_POINT('Origin',(-0.0031262178069016,0.00227581852804816,
0.05925000000001));
#106727=CARTESIAN_POINT('Origin',(-0.00312621780689159,0.00227581852803817,
0.06235));
#106728=CARTESIAN_POINT('',(-0.00307486575549354,0.0157757208597892,0.06235));
#106729=CARTESIAN_POINT('',(-0.00307486575549354,0.0157757208597892,0.05925));
#106730=CARTESIAN_POINT('',(-0.00307486575550355,0.0157757208597992,0.0640296944304424));
#106731=CARTESIAN_POINT('',(-0.0033993108344085,0.015773056030517,0.05925));
#106732=CARTESIAN_POINT('Origin',(-0.0031262178069016,0.00227581852804816,
0.05925000000001));
#106733=CARTESIAN_POINT('',(-0.0033993108344085,0.015773056030517,0.06235));
#106734=CARTESIAN_POINT('',(-0.00339931083441851,0.015773056030527,0.0640346847097368));
#106735=CARTESIAN_POINT('Origin',(-0.0031262178069016,0.00227581852804816,
0.06235000000001));
#106736=CARTESIAN_POINT('Origin',(-0.00312621780689159,0.00227581852803817,
0.06235));
#106737=CARTESIAN_POINT('',(-0.0050558933738229,0.0156371939140674,0.06235));
#106738=CARTESIAN_POINT('',(-0.0050558933738229,0.0156371939140674,0.05925));
#106739=CARTESIAN_POINT('',(-0.0050558933738329,0.0156371939140774,0.0640589676062857));
#106740=CARTESIAN_POINT('',(-0.00473423489955992,0.0156797090464543,0.06235));
#106741=CARTESIAN_POINT('Origin',(-0.0031262178069016,0.00227581852804816,
0.06235000000001));
#106742=CARTESIAN_POINT('',(-0.00473423489955992,0.0156797090464543,0.05925));
#106743=CARTESIAN_POINT('',(-0.00473423489956992,0.0156797090464643,0.0640346847097368));
#106744=CARTESIAN_POINT('Origin',(-0.0031262178069016,0.00227581852804816,
0.05925000000001));
#106745=CARTESIAN_POINT('Origin',(-0.00312621780689159,0.00227581852803817,
0.06235));
#106746=CARTESIAN_POINT('',(-0.000930343506396564,0.0145814325337034,0.06235));
#106747=CARTESIAN_POINT('',(-9.89011778240814E-5,0.0154320092391663,0.06235000000001));
#106748=CARTESIAN_POINT('',(-0.000930343506406564,0.0145814325337134,0.06235000000001));
#106749=CARTESIAN_POINT('',(-0.00245920298515479,0.014758009490669,0.06235));
#106750=CARTESIAN_POINT('',(-0.00173858848308247,0.0157043137847654,0.06235000000001));
#106751=CARTESIAN_POINT('',(-0.00245920298516479,0.014758009490679,0.06235000000001));
#106752=CARTESIAN_POINT('',(-0.00399817372869307,0.014745369156286,0.06235));
#106753=CARTESIAN_POINT('',(-0.00339931083441851,0.015773056030527,0.06235000000001));
#106754=CARTESIAN_POINT('',(-0.00399817372870308,0.014745369156296,0.06235000000001));
#106755=CARTESIAN_POINT('',(-0.0055239265092796,0.0145437031451387,0.06235));
#106756=CARTESIAN_POINT('',(-0.0050558933738329,0.0156371939140774,0.06235000000001));
#106757=CARTESIAN_POINT('',(-0.0055239265092896,0.0145437031451487,0.06235000000001));
#106758=CARTESIAN_POINT('',(-0.00701333247002777,0.0141560685083892,0.06235));
#106759=CARTESIAN_POINT('',(-0.00668322399865577,0.0152987869666117,0.06235000000001));
#106760=CARTESIAN_POINT('',(-0.00701333247003777,0.0141560685083992,0.06235000000001));
#106761=CARTESIAN_POINT('',(-0.0084438137347893,0.0135883413919976,0.06235));
#106762=CARTESIAN_POINT('',(-0.0082566340354241,0.0147629650925005,0.06235000000001));
#106763=CARTESIAN_POINT('',(-0.0084438137347993,0.0135883413920076,0.06235000000001));
#106764=CARTESIAN_POINT('',(-0.00979368566574272,0.0128491279603392,0.06235));
#106765=CARTESIAN_POINT('',(-0.00975227219182637,0.0140378508051684,0.06235000000001));
#106766=CARTESIAN_POINT('',(-0.00979368566575272,0.0128491279603492,0.06235000000001));
#106767=CARTESIAN_POINT('',(-0.0110424855803985,0.0119496339355254,0.06235));
#106768=CARTESIAN_POINT('',(-0.0111474661179811,0.0131344360980708,0.06235000000001));
#106769=CARTESIAN_POINT('',(-0.0110424855804085,0.0119496339355354,0.06235000000001));
#106770=CARTESIAN_POINT('',(-0.0121712829450069,0.0109034947300784,0.06235));
#106771=CARTESIAN_POINT('',(-0.0124210660961502,0.0120664158172769,0.06235000000001));
#106772=CARTESIAN_POINT('',(-0.0121712829450169,0.0109034947300884,0.06235000000001));
#106773=CARTESIAN_POINT('',(-0.0131629663421532,0.00972656874797738,0.06235));
#106774=CARTESIAN_POINT('',(-0.0135537656489009,0.0108499800615636,0.06235000000001));
#106775=CARTESIAN_POINT('',(-0.0131629663421632,0.00972656874798738,0.06235000000001));
#106776=CARTESIAN_POINT('',(-0.014002502862403,0.00843669698741865,0.06235));
#106777=CARTESIAN_POINT('',(-0.0145283942056239,0.00950356875702119,0.06235000000001));
#106778=CARTESIAN_POINT('',(-0.014002502862413,0.00843669698742865,0.06235000000001));
#106779=CARTESIAN_POINT('',(-0.0146771659878858,0.00705343258946943,0.06235));
#106780=CARTESIAN_POINT('',(-0.0153301773908809,0.0080475921265705,0.06235000000001));
#106781=CARTESIAN_POINT('',(-0.0146771659878958,0.00705343258947943,0.06235000000001));
#106782=CARTESIAN_POINT('',(-0.015176728513333,0.00559774443238052,0.06235));
#106783=CARTESIAN_POINT('',(-0.0159469609888762,0.00650412129178826,0.06235000000001));
#106784=CARTESIAN_POINT('',(-0.015176728513343,0.00559774443239052,0.06235000000001));
#106785=CARTESIAN_POINT('',(-0.0154936175800848,0.00409169926476658,0.06235));
#106786=CARTESIAN_POINT('',(-0.0163693951889787,0.00489655369720221,0.06235000000001));
#106787=CARTESIAN_POINT('',(-0.0154936175800948,0.00409169926477658,0.06235000000001));
#106788=CARTESIAN_POINT('',(-0.0156230294729081,0.00255812719619073,0.06235));
#106789=CARTESIAN_POINT('',(-0.0165910763193207,0.00324925842888212,0.06235000000001));
#106790=CARTESIAN_POINT('',(-0.0156230294729181,0.00255812719620073,0.06235000000001));
#106791=CARTESIAN_POINT('',(-0.015563002439423,0.00102027561597532,0.06235));
#106792=CARTESIAN_POINT('',(-0.0166086439199353,0.00158720680393539,0.06235000000001));
#106793=CARTESIAN_POINT('',(-0.015563002439433,0.00102027561598532,0.06235000000001));
#106794=CARTESIAN_POINT('',(-0.0153144464282689,-0.0004985432135232,0.06235));
#106795=CARTESIAN_POINT('',(-0.0164218316839049,-6.44061692259324E-5,0.06235000000001));
#106796=CARTESIAN_POINT('',(-0.0153144464282789,-0.0004985432135332,0.06235000000001));
#106797=CARTESIAN_POINT('',(-0.0148811292952109,-0.00197530554704829,0.06235));
#106798=CARTESIAN_POINT('',(-0.0160334714943015,-0.00168054372145059,0.06235000000001));
#106799=CARTESIAN_POINT('',(-0.0148811292952209,-0.00197530554705829,0.06235000000001));
#106800=CARTESIAN_POINT('',(-0.0142696196862869,-0.00338762517295234,0.06235));
#106801=CARTESIAN_POINT('',(-0.0154494504957272,-0.00323670685486675,0.06235000000001));
#106802=CARTESIAN_POINT('',(-0.0142696196862969,-0.00338762517296234,0.06235000000001));
#106803=CARTESIAN_POINT('',(-0.0134891874638297,-0.004714092765346,0.06235));
#106804=CARTESIAN_POINT('',(-0.0146786218512019,-0.00470930572263721,0.06235000000001));
#106805=CARTESIAN_POINT('',(-0.0134891874638397,-0.004714092765356,0.06235000000001));
#106806=CARTESIAN_POINT('',(-0.012551663184803,-0.0059346004276552,0.06235));
#106807=CARTESIAN_POINT('',(-0.0137326705372373,-0.00607601722701116,0.06235000000001));
#106808=CARTESIAN_POINT('',(-0.012551663184813,-0.0059346004276652,0.06235000000001));
#106809=CARTESIAN_POINT('',(-0.0114712587616171,-0.00703064650783633,0.06235));
#106810=CARTESIAN_POINT('',(-0.0126259362115035,-0.00731612341473131,0.06235000000001));
#106811=CARTESIAN_POINT('',(-0.0114712587616271,-0.00703064650784633,0.06235000000001));
#106812=CARTESIAN_POINT('',(-0.0102643520240239,-0.0079856160645617,0.06235));
#106813=CARTESIAN_POINT('',(-0.0113751958382356,-0.00841082554008646,0.06235000000001));
#106814=CARTESIAN_POINT('',(-0.0102643520240339,-0.0079856160645717,0.06235000000001));
#106815=CARTESIAN_POINT('',(-0.00894923844791235,-0.00878503273279372,0.06235));
#106816=CARTESIAN_POINT('',(-0.00999940936655784,-0.00934352903473414,0.06235000000001));
#106817=CARTESIAN_POINT('',(-0.00894923844792235,-0.00878503273280372,0.06235000000001));
#106818=CARTESIAN_POINT('',(-0.00754585381454333,-0.00941677817072247,0.06235));
#106819=CARTESIAN_POINT('',(-0.00851943231698142,-0.0101000950644411,0.06235000000001));
#106820=CARTESIAN_POINT('',(-0.00754585381455333,-0.00941677817073247,0.06235000000001));
#106821=CARTESIAN_POINT('',(-0.00607547200442719,-0.00987127576147481,0.06235));
#106822=CARTESIAN_POINT('',(-0.00695769963297234,-0.0106690548593978,0.06235000000001));
#106823=CARTESIAN_POINT('',(-0.00607547200443719,-0.00987127576148481,0.06235000000001));
#106824=CARTESIAN_POINT('',(-0.0045603825069806,-0.0101416357848642,0.06235));
#106825=CARTESIAN_POINT('',(-0.00533788559007755,-0.0110417835690786,0.06235000000001));
#106826=CARTESIAN_POINT('',(-0.0045603825069906,-0.0101416357848742,0.06235000000001));
#106827=CARTESIAN_POINT('',(-0.00302355253458767,-0.010223759858526,0.06235));
#106828=CARTESIAN_POINT('',(-0.00368454491803983,-0.0112126310061832,0.06235000000001));
#106829=CARTESIAN_POINT('',(-0.00302355253459767,-0.010223759858536,0.06235000000001));
#106830=CARTESIAN_POINT('',(-0.00148827886307164,-0.0101164030652161,0.06235));
#106831=CARTESIAN_POINT('',(-0.00202274057612456,-0.0111790072977176,0.06235000000001));
#106832=CARTESIAN_POINT('',(-0.00148827886308164,-0.0101164030652261,0.06235000000001));
#106833=CARTESIAN_POINT('',(2.21653236791089E-5,-0.00982119282448763,0.06235));
#106834=CARTESIAN_POINT('',(-0.000377663824205095,-0.010941422144828,0.06235000000001));
#106835=CARTESIAN_POINT('',(2.21653236891089E-5,-0.00982119282449763,0.06235000000001));
#106836=CARTESIAN_POINT('',(0.00148488323145545,-0.00934260422266922,0.06235));
#106837=CARTESIAN_POINT('',(0.00122574765107832,-0.0105034770962511,0.06235000000001));
#106838=CARTESIAN_POINT('',(0.00148488323146545,-0.00934260422267922,0.06235000000001));
#106839=CARTESIAN_POINT('',(0.00287770154778802,-0.00868789217511811,0.06235));
#106840=CARTESIAN_POINT('',(0.0027631877661484,-0.00987181095250685,0.06235000000001));
#106841=CARTESIAN_POINT('',(0.00287770154779802,-0.00868789217512811,0.06235000000001));
#106842=CARTESIAN_POINT('',(0.00417950656676206,-0.00786698144909848,0.06235));
#106843=CARTESIAN_POINT('',(0.00421135049606079,-0.00905599912844934,0.06235000000001));
#106844=CARTESIAN_POINT('',(0.00417950656677206,-0.00786698144910848,0.06235000000001));
#106845=CARTESIAN_POINT('',(0.00537056425127688,-0.00689231621442642,0.06235));
#106846=CARTESIAN_POINT('',(0.00554828317000589,-0.00806840849973849,0.06235000000001));
#106847=CARTESIAN_POINT('',(0.00537056425128688,-0.00689231621443642,0.06235000000001));
#106848=CARTESIAN_POINT('',(0.00643281938093257,-0.00577867140254061,0.06235));
#106849=CARTESIAN_POINT('',(0.00675371925144076,-0.00692400993361114,0.06235000000001));
#106850=CARTESIAN_POINT('',(0.00643281938094257,-0.00577867140255061,0.06235000000001));
#106851=CARTESIAN_POINT('',(0.00735016925076682,-0.00454292873360213,0.06235));
#106852=CARTESIAN_POINT('',(0.00780938555812477,-0.00564015134579409,0.06235000000001));
#106853=CARTESIAN_POINT('',(0.00735016925077682,-0.00454292873361213,0.06235000000001));
#106854=CARTESIAN_POINT('',(0.00810870777184792,-0.00320382080682545,0.06235));
#106855=CARTESIAN_POINT('',(0.00869927926493554,-0.00423629472378529,0.06235000000001));
#106856=CARTESIAN_POINT('',(0.00810870777185792,-0.00320382080683544,0.06235000000001));
#106857=CARTESIAN_POINT('',(0.00869693627340787,-0.00178164713336899,0.06235));
#106858=CARTESIAN_POINT('',(0.00940991049038555,-0.00273372110296171,0.06235000000001));
#106859=CARTESIAN_POINT('',(0.00869693627341787,-0.00178164713337899,0.06235000000001));
#106860=CARTESIAN_POINT('',(0.00910593781097012,-0.000297966416438346,0.06235));
#106861=CARTESIAN_POINT('',(0.00993050678947452,-0.00115520796777584,0.06235000000001));
#106862=CARTESIAN_POINT('',(0.00910593781098012,-0.000297966416448346,0.06235000000001));
#106863=CARTESIAN_POINT('',(0.00932951233813846,0.00122473025667865,0.06235));
#106864=CARTESIAN_POINT('',(0.0102531764529749,0.000475316031710583,0.06235000000001));
#106865=CARTESIAN_POINT('',(0.00932951233814846,0.00122473025668865,0.06235000000001));
#106866=CARTESIAN_POINT('',(0.00936427069298033,0.00276336035656906,0.06235));
#106867=CARTESIAN_POINT('',(0.0103730281376995,0.00213313381369029,0.06235000000001));
#106868=CARTESIAN_POINT('',(0.00936427069299033,0.00276336035657905,0.06235000000001));
#106869=CARTESIAN_POINT('',(0.00920968597426703,0.0042945998193117,0.06235));
#106870=CARTESIAN_POINT('',(0.0102882450142778,0.00379311455049486,0.06235000000001));
#106871=CARTESIAN_POINT('',(0.00920968597427703,0.0042945998193217,0.06235000000001));
#106872=CARTESIAN_POINT('',(0.0088681015287593,0.005795236615511,0.06235));
#106873=CARTESIAN_POINT('',(0.0100001123084378,0.00543009462624556,0.06235000000001));
#106874=CARTESIAN_POINT('',(0.0088681015287693,0.005795236615521,0.06235000000001));
#106875=CARTESIAN_POINT('',(0.00834469542845901,0.00724252262100145,0.06235));
#106876=CARTESIAN_POINT('',(0.00951299781829371,0.00701925909163959,0.06235000000001));
#106877=CARTESIAN_POINT('',(0.00834469542846901,0.00724252262101145,0.06235000000001));
#106878=CARTESIAN_POINT('',(0.0076474019763159,0.00861451845522197,0.06235));
#106879=CARTESIAN_POINT('',(0.00883428570297895,0.00853651783328664,0.06235000000001));
#106880=CARTESIAN_POINT('',(0.0076474019763259,0.00861451845523197,0.06235000000001));
#106881=CARTESIAN_POINT('',(0.00678679143028267,0.00989042605986129,0.06235));
#106882=CARTESIAN_POINT('',(0.00797426454632066,0.00995887075527175,0.06235000000001));
#106883=CARTESIAN_POINT('',(0.00678679143029267,0.00989042605987129,0.06235000000001));
#106884=CARTESIAN_POINT('',(0.0057759097689791,0.0110509039762217,0.06235));
#106885=CARTESIAN_POINT('',(0.00694597139239648,0.0112647564371643,0.06235000000001));
#106886=CARTESIAN_POINT('',(0.0057759097689891,0.0110509039762317,0.06235000000001));
#106887=CARTESIAN_POINT('',(0.00463008092795451,0.0120783605420172,0.06235));
#106888=CARTESIAN_POINT('',(0.00576499411723559,0.0124343789831735,0.06235000000001));
#106889=CARTESIAN_POINT('',(0.00463008092796451,0.0120783605420272,0.06235000000001));
#106890=CARTESIAN_POINT('',(0.00336667450444523,0.0129572205630419,0.06235));
#106891=CARTESIAN_POINT('',(0.00444923513250745,0.0134500081077493,0.06235000000001));
#106892=CARTESIAN_POINT('',(0.00336667450445523,0.0129572205630519,0.06235000000001));
#106893=CARTESIAN_POINT('',(0.00200484245198608,0.0136741614172377,0.06235));
#106894=CARTESIAN_POINT('',(0.00301864000320971,0.0142962479086385,0.06235000000001));
#106895=CARTESIAN_POINT('',(0.00200484245199608,0.0136741614172477,0.06235000000001));
#106896=CARTESIAN_POINT('',(0.000565228756317156,0.0142183150120642,0.06235));
#106897=CARTESIAN_POINT('',(0.00149489509323412,0.014960270253069,0.06235000000001));
#106898=CARTESIAN_POINT('',(0.000565228756327156,0.0142183150120742,0.06235000000001));
#106899=CARTESIAN_POINT('Origin',(-0.00312621780689159,0.00227581852803817,
0.05925));
#106900=CARTESIAN_POINT('',(-0.000930343506396564,0.0145814325337034,0.05925));
#106901=CARTESIAN_POINT('',(-0.000930343506406564,0.0145814325337134,0.05925000000001));
#106902=CARTESIAN_POINT('',(-9.89011778240814E-5,0.0154320092391663,0.05925000000001));
#106903=CARTESIAN_POINT('',(0.000565228756317156,0.0142183150120642,0.05925));
#106904=CARTESIAN_POINT('',(0.000565228756327156,0.0142183150120742,0.05925000000001));
#106905=CARTESIAN_POINT('',(0.00149489509323412,0.014960270253069,0.05925000000001));
#106906=CARTESIAN_POINT('',(0.00200484245198608,0.0136741614172377,0.05925));
#106907=CARTESIAN_POINT('',(0.00200484245199608,0.0136741614172477,0.05925000000001));
#106908=CARTESIAN_POINT('',(0.00301864000320971,0.0142962479086385,0.05925000000001));
#106909=CARTESIAN_POINT('',(0.00336667450444523,0.0129572205630419,0.05925));
#106910=CARTESIAN_POINT('',(0.00336667450445523,0.0129572205630519,0.05925000000001));
#106911=CARTESIAN_POINT('',(0.00444923513250745,0.0134500081077493,0.05925000000001));
#106912=CARTESIAN_POINT('',(0.00463008092795451,0.0120783605420172,0.05925));
#106913=CARTESIAN_POINT('',(0.00463008092796451,0.0120783605420272,0.05925000000001));
#106914=CARTESIAN_POINT('',(0.00576499411723559,0.0124343789831735,0.05925000000001));
#106915=CARTESIAN_POINT('',(0.0057759097689791,0.0110509039762217,0.05925));
#106916=CARTESIAN_POINT('',(0.0057759097689891,0.0110509039762317,0.05925000000001));
#106917=CARTESIAN_POINT('',(0.00694597139239648,0.0112647564371643,0.05925000000001));
#106918=CARTESIAN_POINT('',(0.00678679143028267,0.00989042605986129,0.05925));
#106919=CARTESIAN_POINT('',(0.00678679143029267,0.00989042605987129,0.05925000000001));
#106920=CARTESIAN_POINT('',(0.00797426454632066,0.00995887075527175,0.05925000000001));
#106921=CARTESIAN_POINT('',(0.0076474019763159,0.00861451845522197,0.05925));
#106922=CARTESIAN_POINT('',(0.0076474019763259,0.00861451845523197,0.05925000000001));
#106923=CARTESIAN_POINT('',(0.00883428570297895,0.00853651783328664,0.05925000000001));
#106924=CARTESIAN_POINT('',(0.00834469542845901,0.00724252262100145,0.05925));
#106925=CARTESIAN_POINT('',(0.00834469542846901,0.00724252262101145,0.05925000000001));
#106926=CARTESIAN_POINT('',(0.00951299781829371,0.00701925909163959,0.05925000000001));
#106927=CARTESIAN_POINT('',(0.0088681015287593,0.005795236615511,0.05925));
#106928=CARTESIAN_POINT('',(0.0088681015287693,0.005795236615521,0.05925000000001));
#106929=CARTESIAN_POINT('',(0.0100001123084378,0.00543009462624556,0.05925000000001));
#106930=CARTESIAN_POINT('',(0.00920968597426703,0.0042945998193117,0.05925));
#106931=CARTESIAN_POINT('',(0.00920968597427703,0.0042945998193217,0.05925000000001));
#106932=CARTESIAN_POINT('',(0.0102882450142778,0.00379311455049486,0.05925000000001));
#106933=CARTESIAN_POINT('',(0.00936427069298033,0.00276336035656906,0.05925));
#106934=CARTESIAN_POINT('',(0.00936427069299033,0.00276336035657905,0.05925000000001));
#106935=CARTESIAN_POINT('',(0.0103730281376995,0.00213313381369029,0.05925000000001));
#106936=CARTESIAN_POINT('',(0.00932951233813846,0.00122473025667865,0.05925));
#106937=CARTESIAN_POINT('',(0.00932951233814846,0.00122473025668865,0.05925000000001));
#106938=CARTESIAN_POINT('',(0.0102531764529749,0.000475316031710583,0.05925000000001));
#106939=CARTESIAN_POINT('',(0.00910593781097012,-0.000297966416438346,0.05925));
#106940=CARTESIAN_POINT('',(0.00910593781098012,-0.000297966416448346,0.05925000000001));
#106941=CARTESIAN_POINT('',(0.00993050678947452,-0.00115520796777584,0.05925000000001));
#106942=CARTESIAN_POINT('',(0.00869693627340787,-0.00178164713336899,0.05925));
#106943=CARTESIAN_POINT('',(0.00869693627341787,-0.00178164713337899,0.05925000000001));
#106944=CARTESIAN_POINT('',(0.00940991049038555,-0.00273372110296171,0.05925000000001));
#106945=CARTESIAN_POINT('',(0.00810870777184792,-0.00320382080682545,0.05925));
#106946=CARTESIAN_POINT('',(0.00810870777185792,-0.00320382080683544,0.05925000000001));
#106947=CARTESIAN_POINT('',(0.00869927926493554,-0.00423629472378529,0.05925000000001));
#106948=CARTESIAN_POINT('',(0.00735016925076682,-0.00454292873360213,0.05925));
#106949=CARTESIAN_POINT('',(0.00735016925077682,-0.00454292873361213,0.05925000000001));
#106950=CARTESIAN_POINT('',(0.00780938555812477,-0.00564015134579409,0.05925000000001));
#106951=CARTESIAN_POINT('',(0.00643281938093257,-0.00577867140254061,0.05925));
#106952=CARTESIAN_POINT('',(0.00643281938094257,-0.00577867140255061,0.05925000000001));
#106953=CARTESIAN_POINT('',(0.00675371925144076,-0.00692400993361114,0.05925000000001));
#106954=CARTESIAN_POINT('',(0.00537056425127688,-0.00689231621442642,0.05925));
#106955=CARTESIAN_POINT('',(0.00537056425128688,-0.00689231621443642,0.05925000000001));
#106956=CARTESIAN_POINT('',(0.00554828317000589,-0.00806840849973849,0.05925000000001));
#106957=CARTESIAN_POINT('',(0.00417950656676206,-0.00786698144909848,0.05925));
#106958=CARTESIAN_POINT('',(0.00417950656677206,-0.00786698144910848,0.05925000000001));
#106959=CARTESIAN_POINT('',(0.00421135049606079,-0.00905599912844934,0.05925000000001));
#106960=CARTESIAN_POINT('',(0.00287770154778802,-0.00868789217511811,0.05925));
#106961=CARTESIAN_POINT('',(0.00287770154779802,-0.00868789217512811,0.05925000000001));
#106962=CARTESIAN_POINT('',(0.0027631877661484,-0.00987181095250685,0.05925000000001));
#106963=CARTESIAN_POINT('',(0.00148488323145545,-0.00934260422266922,0.05925));
#106964=CARTESIAN_POINT('',(0.00148488323146545,-0.00934260422267922,0.05925000000001));
#106965=CARTESIAN_POINT('',(0.00122574765107832,-0.0105034770962511,0.05925000000001));
#106966=CARTESIAN_POINT('',(2.21653236791089E-5,-0.00982119282448763,0.05925));
#106967=CARTESIAN_POINT('',(2.21653236891089E-5,-0.00982119282449763,0.05925000000001));
#106968=CARTESIAN_POINT('',(-0.000377663824205095,-0.010941422144828,0.05925000000001));
#106969=CARTESIAN_POINT('',(-0.00148827886307164,-0.0101164030652161,0.05925));
#106970=CARTESIAN_POINT('',(-0.00148827886308164,-0.0101164030652261,0.05925000000001));
#106971=CARTESIAN_POINT('',(-0.00202274057612456,-0.0111790072977176,0.05925000000001));
#106972=CARTESIAN_POINT('',(-0.00302355253458767,-0.010223759858526,0.05925));
#106973=CARTESIAN_POINT('',(-0.00302355253459767,-0.010223759858536,0.05925000000001));
#106974=CARTESIAN_POINT('',(-0.00368454491803983,-0.0112126310061832,0.05925000000001));
#106975=CARTESIAN_POINT('',(-0.0045603825069806,-0.0101416357848642,0.05925));
#106976=CARTESIAN_POINT('',(-0.0045603825069906,-0.0101416357848742,0.05925000000001));
#106977=CARTESIAN_POINT('',(-0.00533788559007755,-0.0110417835690786,0.05925000000001));
#106978=CARTESIAN_POINT('',(-0.00607547200442719,-0.00987127576147481,0.05925));
#106979=CARTESIAN_POINT('',(-0.00607547200443719,-0.00987127576148481,0.05925000000001));
#106980=CARTESIAN_POINT('',(-0.00695769963297234,-0.0106690548593978,0.05925000000001));
#106981=CARTESIAN_POINT('',(-0.00754585381454333,-0.00941677817072247,0.05925));
#106982=CARTESIAN_POINT('',(-0.00754585381455333,-0.00941677817073247,0.05925000000001));
#106983=CARTESIAN_POINT('',(-0.00851943231698142,-0.0101000950644411,0.05925000000001));
#106984=CARTESIAN_POINT('',(-0.00894923844791235,-0.00878503273279372,0.05925));
#106985=CARTESIAN_POINT('',(-0.00894923844792235,-0.00878503273280372,0.05925000000001));
#106986=CARTESIAN_POINT('',(-0.00999940936655784,-0.00934352903473414,0.05925000000001));
#106987=CARTESIAN_POINT('',(-0.0102643520240239,-0.0079856160645617,0.05925));
#106988=CARTESIAN_POINT('',(-0.0102643520240339,-0.0079856160645717,0.05925000000001));
#106989=CARTESIAN_POINT('',(-0.0113751958382356,-0.00841082554008646,0.05925000000001));
#106990=CARTESIAN_POINT('',(-0.0114712587616171,-0.00703064650783633,0.05925));
#106991=CARTESIAN_POINT('',(-0.0114712587616271,-0.00703064650784633,0.05925000000001));
#106992=CARTESIAN_POINT('',(-0.0126259362115035,-0.00731612341473131,0.05925000000001));
#106993=CARTESIAN_POINT('',(-0.012551663184803,-0.0059346004276552,0.05925));
#106994=CARTESIAN_POINT('',(-0.012551663184813,-0.0059346004276652,0.05925000000001));
#106995=CARTESIAN_POINT('',(-0.0137326705372373,-0.00607601722701116,0.05925000000001));
#106996=CARTESIAN_POINT('',(-0.0134891874638297,-0.004714092765346,0.05925));
#106997=CARTESIAN_POINT('',(-0.0134891874638397,-0.004714092765356,0.05925000000001));
#106998=CARTESIAN_POINT('',(-0.0146786218512019,-0.00470930572263721,0.05925000000001));
#106999=CARTESIAN_POINT('',(-0.0142696196862869,-0.00338762517295234,0.05925));
#107000=CARTESIAN_POINT('',(-0.0142696196862969,-0.00338762517296234,0.05925000000001));
#107001=CARTESIAN_POINT('',(-0.0154494504957272,-0.00323670685486675,0.05925000000001));
#107002=CARTESIAN_POINT('',(-0.0148811292952109,-0.00197530554704829,0.05925));
#107003=CARTESIAN_POINT('',(-0.0148811292952209,-0.00197530554705829,0.05925000000001));
#107004=CARTESIAN_POINT('',(-0.0160334714943015,-0.00168054372145059,0.05925000000001));
#107005=CARTESIAN_POINT('',(-0.0153144464282689,-0.0004985432135232,0.05925));
#107006=CARTESIAN_POINT('',(-0.0153144464282789,-0.0004985432135332,0.05925000000001));
#107007=CARTESIAN_POINT('',(-0.0164218316839049,-6.44061692259324E-5,0.05925000000001));
#107008=CARTESIAN_POINT('',(-0.015563002439423,0.00102027561597532,0.05925));
#107009=CARTESIAN_POINT('',(-0.015563002439433,0.00102027561598532,0.05925000000001));
#107010=CARTESIAN_POINT('',(-0.0166086439199353,0.00158720680393539,0.05925000000001));
#107011=CARTESIAN_POINT('',(-0.0156230294729081,0.00255812719619073,0.05925));
#107012=CARTESIAN_POINT('',(-0.0156230294729181,0.00255812719620073,0.05925000000001));
#107013=CARTESIAN_POINT('',(-0.0165910763193207,0.00324925842888212,0.05925000000001));
#107014=CARTESIAN_POINT('',(-0.0154936175800848,0.00409169926476658,0.05925));
#107015=CARTESIAN_POINT('',(-0.0154936175800948,0.00409169926477658,0.05925000000001));
#107016=CARTESIAN_POINT('',(-0.0163693951889787,0.00489655369720221,0.05925000000001));
#107017=CARTESIAN_POINT('',(-0.015176728513333,0.00559774443238052,0.05925));
#107018=CARTESIAN_POINT('',(-0.015176728513343,0.00559774443239052,0.05925000000001));
#107019=CARTESIAN_POINT('',(-0.0159469609888762,0.00650412129178826,0.05925000000001));
#107020=CARTESIAN_POINT('',(-0.0146771659878858,0.00705343258946943,0.05925));
#107021=CARTESIAN_POINT('',(-0.0146771659878958,0.00705343258947943,0.05925000000001));
#107022=CARTESIAN_POINT('',(-0.0153301773908809,0.0080475921265705,0.05925000000001));
#107023=CARTESIAN_POINT('',(-0.014002502862403,0.00843669698741865,0.05925));
#107024=CARTESIAN_POINT('',(-0.014002502862413,0.00843669698742865,0.05925000000001));
#107025=CARTESIAN_POINT('',(-0.0145283942056239,0.00950356875702119,0.05925000000001));
#107026=CARTESIAN_POINT('',(-0.0131629663421532,0.00972656874797738,0.05925));
#107027=CARTESIAN_POINT('',(-0.0131629663421632,0.00972656874798738,0.05925000000001));
#107028=CARTESIAN_POINT('',(-0.0135537656489009,0.0108499800615636,0.05925000000001));
#107029=CARTESIAN_POINT('',(-0.0121712829450069,0.0109034947300784,0.05925));
#107030=CARTESIAN_POINT('',(-0.0121712829450169,0.0109034947300884,0.05925000000001));
#107031=CARTESIAN_POINT('',(-0.0124210660961502,0.0120664158172769,0.05925000000001));
#107032=CARTESIAN_POINT('',(-0.0110424855803985,0.0119496339355254,0.05925));
#107033=CARTESIAN_POINT('',(-0.0110424855804085,0.0119496339355354,0.05925000000001));
#107034=CARTESIAN_POINT('',(-0.0111474661179811,0.0131344360980708,0.05925000000001));
#107035=CARTESIAN_POINT('',(-0.00979368566574272,0.0128491279603392,0.05925));
#107036=CARTESIAN_POINT('',(-0.00979368566575272,0.0128491279603492,0.05925000000001));
#107037=CARTESIAN_POINT('',(-0.00975227219182637,0.0140378508051684,0.05925000000001));
#107038=CARTESIAN_POINT('',(-0.0084438137347893,0.0135883413919976,0.05925));
#107039=CARTESIAN_POINT('',(-0.0084438137347993,0.0135883413920076,0.05925000000001));
#107040=CARTESIAN_POINT('',(-0.0082566340354241,0.0147629650925005,0.05925000000001));
#107041=CARTESIAN_POINT('',(-0.00701333247002777,0.0141560685083892,0.05925));
#107042=CARTESIAN_POINT('',(-0.00701333247003777,0.0141560685083992,0.05925000000001));
#107043=CARTESIAN_POINT('',(-0.00668322399865577,0.0152987869666117,0.05925000000001));
#107044=CARTESIAN_POINT('',(-0.0055239265092796,0.0145437031451387,0.05925));
#107045=CARTESIAN_POINT('',(-0.0055239265092896,0.0145437031451487,0.05925000000001));
#107046=CARTESIAN_POINT('',(-0.0050558933738329,0.0156371939140774,0.05925000000001));
#107047=CARTESIAN_POINT('',(-0.00399817372869307,0.014745369156286,0.05925));
#107048=CARTESIAN_POINT('',(-0.00399817372870308,0.014745369156296,0.05925000000001));
#107049=CARTESIAN_POINT('',(-0.00339931083441851,0.015773056030527,0.05925000000001));
#107050=CARTESIAN_POINT('',(-0.00245920298515479,0.014758009490669,0.05925));
#107051=CARTESIAN_POINT('',(-0.00245920298516479,0.014758009490679,0.05925000000001));
#107052=CARTESIAN_POINT('',(-0.00173858848308247,0.0157043137847654,0.05925000000001));
#107053=CARTESIAN_POINT('Origin',(-0.00312621780689159,0.00227581852803817,
0.05991));
#107054=CARTESIAN_POINT('Origin',(-0.00312621780689159,0.00227581852803817,
0.06169));
#107055=CARTESIAN_POINT('Origin',(-0.00312621780689159,0.00227581852803817,
0.06603));
#107056=CARTESIAN_POINT('Origin',(-0.00312621780689159,0.00227581852803817,
0.05925));
#107057=CARTESIAN_POINT('Origin',(-0.00399817372869307,0.014745369156286,
0.0640346847097268));
#107058=CARTESIAN_POINT('',(-0.00399817372870308,0.014745369156296,0.0640346847097368));
#107059=CARTESIAN_POINT('Origin',(-0.0033993108344085,0.015773056030517,
0.0640346847097268));
#107060=CARTESIAN_POINT('Origin',(-0.00245920298515479,0.014758009490669,
0.0640296944304324));
#107061=CARTESIAN_POINT('',(-0.00245920298516479,0.014758009490679,0.0640296944304424));
#107062=CARTESIAN_POINT('Origin',(-0.00173858848307247,0.0157043137847554,
0.0640296944304324));
#107063=CARTESIAN_POINT('Origin',(-0.0055239265092796,0.0145437031451387,
0.0640589676062757));
#107064=CARTESIAN_POINT('',(-0.0055239265092896,0.0145437031451487,0.0640589676062857));
#107065=CARTESIAN_POINT('Origin',(-0.0050558933738229,0.0156371939140674,
0.0640589676062757));
#107066=CARTESIAN_POINT('Origin',(-0.0146771659878858,0.00705343258946943,
0.0640485717989425));
#107067=CARTESIAN_POINT('',(-0.0146771659878958,0.00705343258947943,0.0640485717989525));
#107068=CARTESIAN_POINT('Origin',(-0.0153301773908709,0.0080475921265605,
0.0640485717989425));
#107069=CARTESIAN_POINT('Origin',(-0.014002502862403,0.00843669698741865,
0.0640116263041342));
#107070=CARTESIAN_POINT('',(-0.014002502862413,0.00843669698742865,0.0640116263041442));
#107071=CARTESIAN_POINT('Origin',(-0.0145283942056139,0.00950356875701119,
0.0640116263041342));
#107072=CARTESIAN_POINT('Origin',(-0.0131629663421532,0.00972656874797738,
0.0639853702628534));
#107073=CARTESIAN_POINT('',(-0.0131629663421632,0.00972656874798738,0.0639853702628634));
#107074=CARTESIAN_POINT('Origin',(-0.0135537656488909,0.0108499800615536,
0.0639853702628534));
#107075=CARTESIAN_POINT('Origin',(-0.0121712829450069,0.0109034947300784,
0.0640020568079285));
#107076=CARTESIAN_POINT('',(-0.0121712829450169,0.0109034947300884,0.0640020568079385));
#107077=CARTESIAN_POINT('Origin',(-0.0124210660961402,0.0120664158172669,
0.0640020568079285));
#107078=CARTESIAN_POINT('Origin',(-0.0110424855803985,0.0119496339355254,
0.0639946102147255));
#107079=CARTESIAN_POINT('',(-0.0110424855804085,0.0119496339355354,0.0639946102147355));
#107080=CARTESIAN_POINT('Origin',(-0.0111474661179711,0.0131344360980608,
0.0639946102147255));
#107081=CARTESIAN_POINT('Origin',(-0.00979368566574272,0.0128491279603392,
0.0639914355303126));
#107082=CARTESIAN_POINT('',(-0.00979368566575272,0.0128491279603492,0.0639914355303226));
#107083=CARTESIAN_POINT('Origin',(-0.00975227219181637,0.0140378508051584,
0.0639914355303126));
#107084=CARTESIAN_POINT('Origin',(-0.0084438137347893,0.0135883413919976,
0.0640371289970071));
#107085=CARTESIAN_POINT('',(-0.0084438137347993,0.0135883413920076,0.0640371289970171));
#107086=CARTESIAN_POINT('Origin',(-0.0082566340354141,0.0147629650924905,
0.0640371289970071));
#107087=CARTESIAN_POINT('Origin',(-0.00701333247002777,0.0141560685083892,
0.0640597876942985));
#107088=CARTESIAN_POINT('',(-0.00701333247003777,0.0141560685083992,0.0640597876943085));
#107089=CARTESIAN_POINT('Origin',(-0.00668322399864577,0.0152987869666017,
0.0640597876942985));
#107090=CARTESIAN_POINT('Origin',(-0.015176728513333,0.00559774443238052,
0.0640622576161347));
#107091=CARTESIAN_POINT('',(-0.015176728513343,0.00559774443239052,0.0640622576161447));
#107092=CARTESIAN_POINT('Origin',(-0.0159469609888662,0.00650412129177826,
0.0640622576161347));
#107093=CARTESIAN_POINT('Origin',(-0.0154936175800848,0.00409169926476658,
0.0640524165708833));
#107094=CARTESIAN_POINT('',(-0.0154936175800948,0.00409169926477658,0.0640524165708933));
#107095=CARTESIAN_POINT('Origin',(-0.0163693951889687,0.00489655369719221,
0.0640524165708833));
#107096=CARTESIAN_POINT('Origin',(-0.0156230294729081,0.00255812719619073,
0.0640221869975658));
#107097=CARTESIAN_POINT('',(-0.0156230294729181,0.00255812719620073,0.0640221869975759));
#107098=CARTESIAN_POINT('Origin',(-0.0165910763193107,0.00324925842887212,
0.0640221869975658));
#107099=CARTESIAN_POINT('Origin',(-0.015563002439423,0.00102027561597532,
0.0640429369448756));
#107100=CARTESIAN_POINT('',(-0.015563002439433,0.00102027561598532,0.0640429369448856));
#107101=CARTESIAN_POINT('Origin',(-0.0166086439199253,0.00158720680392539,
0.0640429369448756));
#107102=CARTESIAN_POINT('Origin',(-0.0153144464282689,-0.0004985432135232,
0.064061380725464));
#107103=CARTESIAN_POINT('',(-0.0153144464282789,-0.0004985432135332,0.064061380725474));
#107104=CARTESIAN_POINT('Origin',(-0.0164218316838949,-6.44061692159324E-5,
0.064061380725464));
#107105=CARTESIAN_POINT('Origin',(-0.0148811292952109,-0.00197530554704829,
0.0640563147052241));
#107106=CARTESIAN_POINT('',(-0.0148811292952209,-0.00197530554705829,0.0640563147052341));
#107107=CARTESIAN_POINT('Origin',(-0.0160334714942915,-0.00168054372144059,
0.0640563147052241));
#107108=CARTESIAN_POINT('Origin',(-0.0142696196862869,-0.00338762517295234,
0.0640278376069354));
#107109=CARTESIAN_POINT('',(-0.0142696196862969,-0.00338762517296234,0.0640278376069454));
#107110=CARTESIAN_POINT('Origin',(-0.0154494504957172,-0.00323670685485675,
0.0640278376069354));
#107111=CARTESIAN_POINT('Origin',(-0.0134891874638297,-0.004714092765346,
0.06397650941055));
#107112=CARTESIAN_POINT('',(-0.0134891874638397,-0.004714092765356,0.06397650941056));
#107113=CARTESIAN_POINT('Origin',(-0.0146786218511919,-0.00470930572262721,
0.06397650941055));
#107114=CARTESIAN_POINT('Origin',(-0.0114712587616171,-0.00703064650783633,
0.0640001436148948));
#107115=CARTESIAN_POINT('',(-0.0114712587616271,-0.00703064650784633,0.0640001436149048));
#107116=CARTESIAN_POINT('Origin',(-0.0126259362114935,-0.00731612341472131,
0.0640001436148948));
#107117=CARTESIAN_POINT('Origin',(-0.012551663184803,-0.0059346004276552,
0.0639987344374606));
#107118=CARTESIAN_POINT('',(-0.012551663184813,-0.0059346004276652,0.0639987344374706));
#107119=CARTESIAN_POINT('Origin',(-0.0137326705372273,-0.00607601722700116,
0.0639987344374606));
#107120=CARTESIAN_POINT('Origin',(-0.0102643520240239,-0.0079856160645617,
0.0639774518569439));
#107121=CARTESIAN_POINT('',(-0.0102643520240339,-0.0079856160645717,0.0639774518569539));
#107122=CARTESIAN_POINT('Origin',(-0.0113751958382256,-0.00841082554007646,
0.0639774518569439));
#107123=CARTESIAN_POINT('Origin',(-0.00894923844791235,-0.00878503273279372,
0.064023011312247));
#107124=CARTESIAN_POINT('',(-0.00894923844792235,-0.00878503273280372,0.064023011312257));
#107125=CARTESIAN_POINT('Origin',(-0.00999940936654784,-0.00934352903472414,
0.064023011312247));
#107126=CARTESIAN_POINT('Origin',(-0.00754585381454333,-0.00941677817072247,
0.0640541921468364));
#107127=CARTESIAN_POINT('',(-0.00754585381455333,-0.00941677817073247,0.0640541921468464));
#107128=CARTESIAN_POINT('Origin',(-0.00851943231697142,-0.0101000950644311,
0.0640541921468364));
#107129=CARTESIAN_POINT('Origin',(-0.00607547200442719,-0.00987127576147481,
0.0640620033446039));
#107130=CARTESIAN_POINT('',(-0.00607547200443719,-0.00987127576148481,0.0640620033446139));
#107131=CARTESIAN_POINT('Origin',(-0.00695769963296234,-0.0106690548593878,
0.0640620033446039));
#107132=CARTESIAN_POINT('Origin',(-0.0045603825069806,-0.0101416357848642,
0.0640462926264731));
#107133=CARTESIAN_POINT('',(-0.0045603825069906,-0.0101416357848742,0.0640462926264831));
#107134=CARTESIAN_POINT('Origin',(-0.00533788559006755,-0.0110417835690686,
0.0640462926264731));
#107135=CARTESIAN_POINT('Origin',(-0.00302355253458767,-0.010223759858526,
0.0640207658501684));
#107136=CARTESIAN_POINT('',(-0.00302355253459767,-0.010223759858536,0.0640207658501784));
#107137=CARTESIAN_POINT('Origin',(-0.00368454491802983,-0.0112126310061732,
0.0640207658501684));
#107138=CARTESIAN_POINT('Origin',(-0.00148827886307164,-0.0101164030652161,
0.0640497400911627));
#107139=CARTESIAN_POINT('',(-0.00148827886308164,-0.0101164030652261,0.0640497400911727));
#107140=CARTESIAN_POINT('Origin',(-0.00202274057611456,-0.0111790072977077,
0.0640497400911627));
#107141=CARTESIAN_POINT('Origin',(2.21653236791089E-5,-0.00982119282448763,
0.0640623222440536));
#107142=CARTESIAN_POINT('',(2.21653236891089E-5,-0.00982119282449763,0.0640623222440636));
#107143=CARTESIAN_POINT('Origin',(-0.000377663824195094,-0.010941422144818,
0.0640623222440536));
#107144=CARTESIAN_POINT('Origin',(0.00148488323145545,-0.00934260422266922,
0.0640513762773474));
#107145=CARTESIAN_POINT('',(0.00148488323146545,-0.00934260422267922,0.0640513762773574));
#107146=CARTESIAN_POINT('Origin',(0.00122574765106832,-0.0105034770962411,
0.0640513762773474));
#107147=CARTESIAN_POINT('Origin',(0.00287770154778802,-0.00868789217511811,
0.0640171157235525));
#107148=CARTESIAN_POINT('',(0.00287770154779802,-0.00868789217512811,0.0640171157235625));
#107149=CARTESIAN_POINT('Origin',(0.00276318776613839,-0.00987181095249685,
0.0640171157235525));
#107150=CARTESIAN_POINT('Origin',(0.00735016925076682,-0.00454292873360213,
0.0639846412562978));
#107151=CARTESIAN_POINT('',(0.00735016925077682,-0.00454292873361213,0.0639846412563078));
#107152=CARTESIAN_POINT('Origin',(0.00780938555811477,-0.00564015134578409,
0.0639846412562978));
#107153=CARTESIAN_POINT('Origin',(0.00643281938093257,-0.00577867140254061,
0.0639967221271682));
#107154=CARTESIAN_POINT('',(0.00643281938094257,-0.00577867140255061,0.0639967221271783));
#107155=CARTESIAN_POINT('Origin',(0.00675371925143076,-0.00692400993360114,
0.0639967221271682));
#107156=CARTESIAN_POINT('Origin',(0.00537056425127688,-0.00689231621442642,
0.064001351848474));
#107157=CARTESIAN_POINT('',(0.00537056425128688,-0.00689231621443642,0.064001351848484));
#107158=CARTESIAN_POINT('Origin',(0.00554828316999589,-0.00806840849972849,
0.064001351848474));
#107159=CARTESIAN_POINT('Origin',(0.00417950656676206,-0.00786698144909848,
0.0639818602956437));
#107160=CARTESIAN_POINT('',(0.00417950656677206,-0.00786698144910848,0.0639818602956537));
#107161=CARTESIAN_POINT('Origin',(0.0042113504960508,-0.00905599912843934,
0.0639818602956437));
#107162=CARTESIAN_POINT('Origin',(0.00810870777184792,-0.00320382080682545,
0.064032971803573));
#107163=CARTESIAN_POINT('',(0.00810870777185792,-0.00320382080683544,0.064032971803583));
#107164=CARTESIAN_POINT('Origin',(0.00869927926492554,-0.00423629472377529,
0.064032971803573));
#107165=CARTESIAN_POINT('Origin',(0.00869693627340787,-0.00178164713336899,
0.0640583496424));
#107166=CARTESIAN_POINT('',(0.00869693627341787,-0.00178164713337899,0.06405834964241));
#107167=CARTESIAN_POINT('Origin',(0.00940991049037555,-0.00273372110295171,
0.0640583496424));
#107168=CARTESIAN_POINT('Origin',(0.00910593781097012,-0.000297966416438346,
0.0640602767162906));
#107169=CARTESIAN_POINT('',(0.00910593781098012,-0.000297966416448346,0.0640602767163006));
#107170=CARTESIAN_POINT('Origin',(0.00993050678946452,-0.00115520796776584,
0.0640602767162906));
#107171=CARTESIAN_POINT('Origin',(0.00932951233813846,0.00122473025667865,
0.0640387154811068));
#107172=CARTESIAN_POINT('',(0.00932951233814846,0.00122473025668865,0.0640387154811168));
#107173=CARTESIAN_POINT('Origin',(0.0102531764529649,0.000475316031700583,
0.0640387154811068));
#107174=CARTESIAN_POINT('Origin',(0.00936427069298033,0.00276336035656906,
0.0640254477644175));
#107175=CARTESIAN_POINT('',(0.00936427069299033,0.00276336035657905,0.0640254477644275));
#107176=CARTESIAN_POINT('Origin',(0.0103730281376895,0.00213313381368028,
0.0640254477644175));
#107177=CARTESIAN_POINT('Origin',(0.00920968597426703,0.0042945998193117,
0.0640550858195568));
#107178=CARTESIAN_POINT('',(0.00920968597427703,0.0042945998193217,0.0640550858195668));
#107179=CARTESIAN_POINT('Origin',(0.0102882450142678,0.00379311455048486,
0.0640550858195568));
#107180=CARTESIAN_POINT('Origin',(0.0088681015287593,0.005795236615511,
0.0640617910186438));
#107181=CARTESIAN_POINT('',(0.0088681015287693,0.005795236615521,0.0640617910186538));
#107182=CARTESIAN_POINT('Origin',(0.0100001123084278,0.00543009462623556,
0.0640617910186438));
#107183=CARTESIAN_POINT('Origin',(0.00834469542845901,0.00724252262100145,
0.064044978432879));
#107184=CARTESIAN_POINT('',(0.00834469542846901,0.00724252262101145,0.064044978432889));
#107185=CARTESIAN_POINT('Origin',(0.00951299781828371,0.00701925909162959,
0.064044978432879));
#107186=CARTESIAN_POINT('Origin',(0.0076474019763159,0.00861451845522197,
0.0640049766461023));
#107187=CARTESIAN_POINT('',(0.0076474019763259,0.00861451845523197,0.0640049766461123));
#107188=CARTESIAN_POINT('Origin',(0.00883428570296894,0.00853651783327664,
0.0640049766461023));
#107189=CARTESIAN_POINT('Origin',(0.00678679143028267,0.00989042605986129,
0.0639889835233511));
#107190=CARTESIAN_POINT('',(0.00678679143029267,0.00989042605987129,0.0639889835233611));
#107191=CARTESIAN_POINT('Origin',(0.00797426454631066,0.00995887075526175,
0.0639889835233511));
#107192=CARTESIAN_POINT('Origin',(0.0057759097689791,0.0110509039762217,
0.0640024596936878));
#107193=CARTESIAN_POINT('',(0.0057759097689891,0.0110509039762317,0.0640024596936978));
#107194=CARTESIAN_POINT('Origin',(0.00694597139238648,0.0112647564371543,
0.0640024596936878));
#107195=CARTESIAN_POINT('Origin',(0.00463008092795451,0.0120783605420172,
0.0639917959462776));
#107196=CARTESIAN_POINT('',(0.00463008092796451,0.0120783605420272,0.0639917959462876));
#107197=CARTESIAN_POINT('Origin',(0.00576499411722559,0.0124343789831635,
0.0639917959462776));
#107198=CARTESIAN_POINT('Origin',(0.00336667450444523,0.0129572205630419,
0.0639988309423512));
#107199=CARTESIAN_POINT('',(0.00336667450445523,0.0129572205630519,0.0639988309423612));
#107200=CARTESIAN_POINT('Origin',(0.00444923513249744,0.0134500081077393,
0.0639988309423512));
#107201=CARTESIAN_POINT('Origin',(0.00200484245198608,0.0136741614172377,
0.0640414954613487));
#107202=CARTESIAN_POINT('',(0.00200484245199608,0.0136741614172477,0.0640414954613587));
#107203=CARTESIAN_POINT('Origin',(0.00301864000319971,0.0142962479086285,
0.0640414954613487));
#107204=CARTESIAN_POINT('Origin',(0.000565228756317156,0.0142183150120642,
0.0640610392221339));
#107205=CARTESIAN_POINT('',(0.000565228756327156,0.0142183150120742,0.0640610392221439));
#107206=CARTESIAN_POINT('Origin',(0.00149489509322412,0.014960270253059,
0.0640610392221339));
#107207=CARTESIAN_POINT('Origin',(-0.000930343506396564,0.0145814325337034,
0.0640570798288145));
#107208=CARTESIAN_POINT('',(-0.000930343506406564,0.0145814325337134,0.0640570798288245));
#107209=CARTESIAN_POINT('Origin',(-9.89011778140814E-5,0.0154320092391563,
0.0640570798288145));
#107896=UNCERTAINTY_MEASURE_WITH_UNIT(LENGTH_MEASURE(1.E-5),#107911,
'DISTANCE_ACCURACY_VALUE',
'Maximum model space distance between geometric entities at asserted c
onnectivities');
#107898=UNCERTAINTY_MEASURE_WITH_UNIT(LENGTH_MEASURE(1.E-5),#107911,
'DISTANCE_ACCURACY_VALUE',
'Maximum model space distance between geometric entities at asserted c
onnectivities');
#107908=(
GEOMETRIC_REPRESENTATION_CONTEXT(3)
GLOBAL_UNCERTAINTY_ASSIGNED_CONTEXT((#107896))
GLOBAL_UNIT_ASSIGNED_CONTEXT((#107911,#107912,#107913))
REPRESENTATION_CONTEXT('','3D')
);
#107910=(
GEOMETRIC_REPRESENTATION_CONTEXT(3)
GLOBAL_UNCERTAINTY_ASSIGNED_CONTEXT((#107898))
GLOBAL_UNIT_ASSIGNED_CONTEXT((#107911,#107912,#107913))
REPRESENTATION_CONTEXT('','3D')
);
#107911=(
LENGTH_UNIT()
NAMED_UNIT(*)
SI_UNIT($,.METRE.)
);
#107912=(
NAMED_UNIT(*)
PLANE_ANGLE_UNIT()
SI_UNIT($,.RADIAN.)
);
#107913=(
NAMED_UNIT(*)
SI_UNIT($,.STERADIAN.)
SOLID_ANGLE_UNIT()
);
#107923=SHAPE_DEFINITION_REPRESENTATION(#107934,#107955);
#107934=PRODUCT_DEFINITION_SHAPE('',$,#107967);
#107955=SHAPE_REPRESENTATION('',(#49899),#107908);
#107957=PRODUCT_DEFINITION_CONTEXT('part definition',#107992,'design');
#107967=PRODUCT_DEFINITION('Gear','Gear',#107978,#107957);
#107978=PRODUCT_DEFINITION_FORMATION('',$,#108003);
#107992=APPLICATION_CONTEXT('Managed model based 3d engineering');
#107993=PRODUCT_CONTEXT('part definition',#107992,'mechanical');
#108003=PRODUCT('Gear','Gear',
'LEGAL AND USAGE DISCLAIMER: this Data/Model is provided \X2\201C\X0\A
S IS\X2\201D\X0\ for informational and representational only. It is a 
geometric approximation and is NOT engineered, certified, or guarantee
d for dimensional accuracy, exact tolerances, or production-level prec
ision. Vendor disclaims all implied warranties including fitness for a
 particular purpose. DO NOT USE FOR DIRECT PHYSICAL MANUFACTURING, AUT
OMATED PRODUCTION, OR SAFETY-CRITICAL SYSTEMS without independent engi
neering verification and resolution of any design discrepancies.',(#107993));
#108006=PRESENTATION_STYLE_ASSIGNMENT((#108013));
#108013=SURFACE_STYLE_USAGE(.BOTH.,#108020);
#108020=SURFACE_SIDE_STYLE('',(#108027));
#108027=SURFACE_STYLE_FILL_AREA(#108034);
#108034=FILL_AREA_STYLE('Opaque(25,25,25)',(#108041));
#108041=FILL_AREA_STYLE_COLOUR('Opaque(25,25,25)',#108048);
#108048=COLOUR_RGB('Opaque(25,25,25)',0.0980392156862745,0.0980392156862745,
0.0980392156862745);
ENDSEC;
END-ISO-10303-21;
